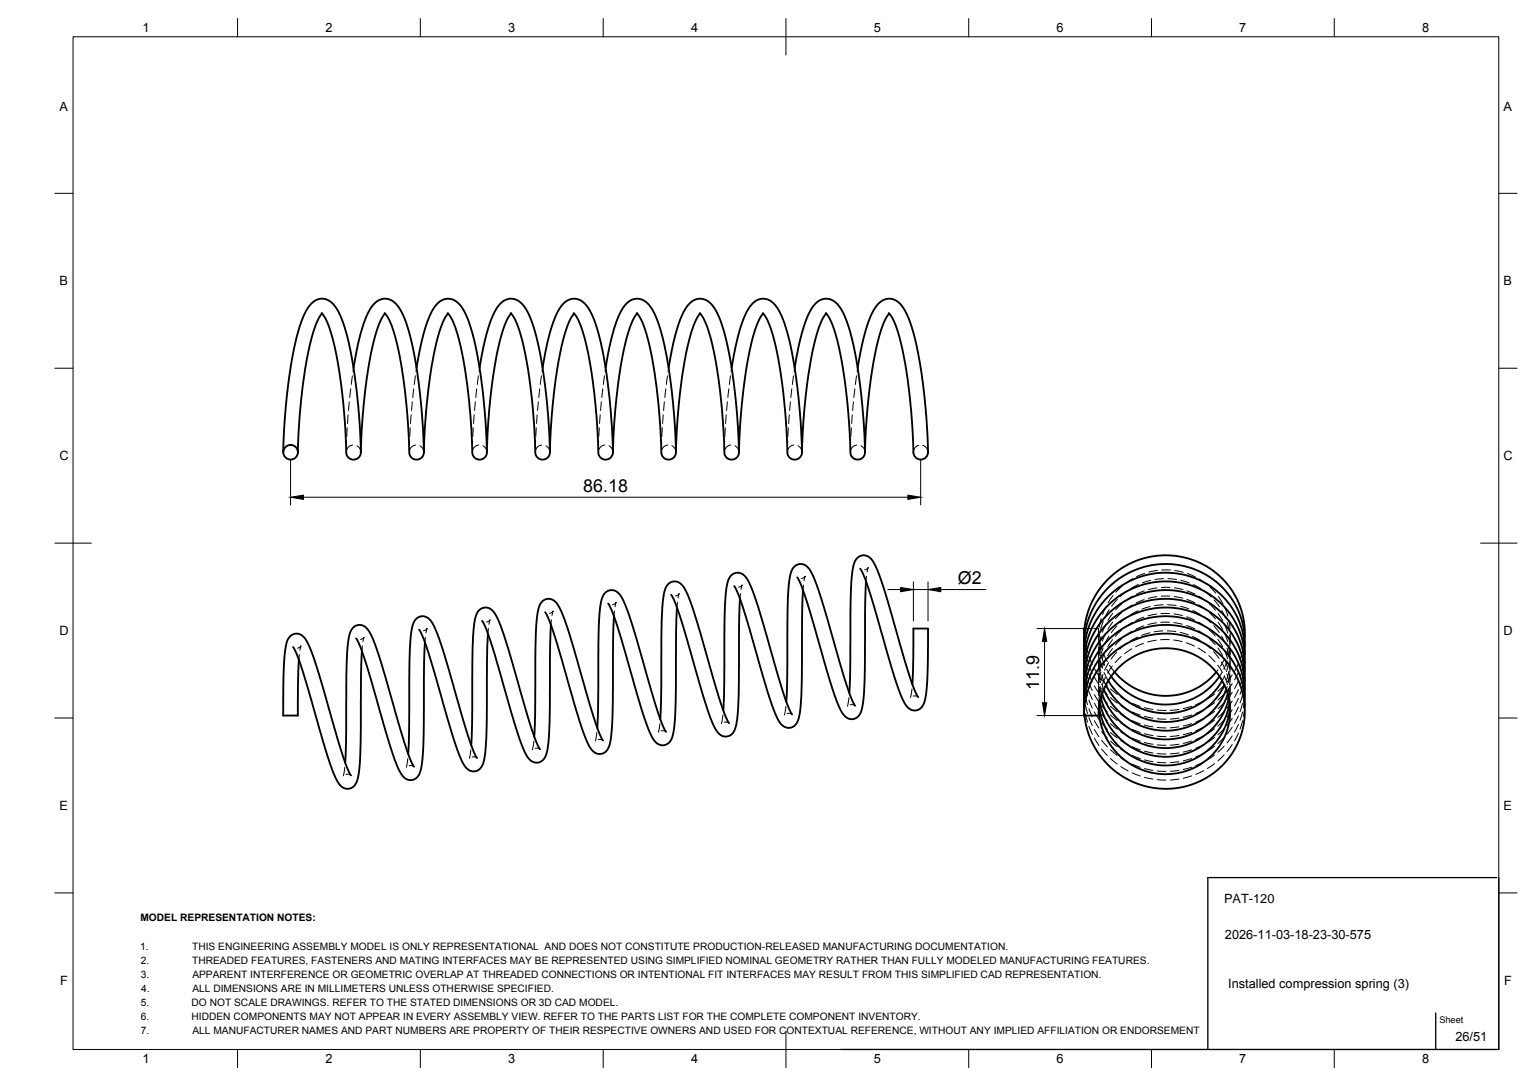
ISO-10303-21;
HEADER;
/* Generated by software containing ST-Developer
 * from STEP Tools, Inc. (www.steptools.com) 
 */

FILE_DESCRIPTION(
/* description */ ('Vibration shaker table dummy'),
/* implementation_level */ '2;1');

FILE_NAME(
/* name */ 'Installed compression spring (3).step',
/* time_stamp */ '2026-10-27T10:55:14-07:00',
/* author */ (''),
/* organization */ (''),
/* preprocessor_version */ 'ST-DEVELOPER v20.2',
/* originating_system */ 'Autodesk Translation Framework v15.17.0.0',
/* authorisation */ '');

FILE_SCHEMA (('AUTOMOTIVE_DESIGN { 1 0 10303 214 3 1 1 }'));
ENDSEC;

DATA;
#10=MECHANICAL_DESIGN_GEOMETRIC_PRESENTATION_REPRESENTATION('',(#707),#22394);
#589=B_SPLINE_CURVE_WITH_KNOTS('',3,(#20705,#20706,#20707,#20708,#20709,
#20710,#20711,#20712,#20713,#20714,#20715,#20716,#20717,#20718,#20719,#20720,
#20721,#20722,#20723,#20724,#20725,#20726,#20727,#20728,#20729,#20730,#20731,
#20732,#20733,#20734,#20735,#20736,#20737,#20738,#20739,#20740,#20741,#20742,
#20743,#20744,#20745,#20746,#20747,#20748,#20749,#20750,#20751,#20752,#20753,
#20754,#20755,#20756,#20757,#20758,#20759,#20760,#20761,#20762,#20763,#20764,
#20765,#20766,#20767,#20768,#20769,#20770,#20771,#20772,#20773,#20774,#20775,
#20776,#20777,#20778,#20779,#20780,#20781,#20782,#20783,#20784,#20785,#20786,
#20787,#20788,#20789,#20790,#20791,#20792,#20793,#20794,#20795,#20796,#20797,
#20798,#20799,#20800,#20801,#20802,#20803,#20804,#20805,#20806,#20807,#20808,
#20809,#20810,#20811,#20812,#20813,#20814,#20815,#20816,#20817,#20818,#20819,
#20820,#20821,#20822,#20823,#20824,#20825,#20826,#20827,#20828,#20829,#20830,
#20831),.UNSPECIFIED.,.F.,.F.,(4,1,1,1,1,1,1,1,1,1,1,1,1,1,1,1,1,1,1,1,
1,1,1,1,1,1,1,1,1,1,1,1,1,1,1,1,1,1,1,1,1,1,1,1,1,1,1,1,1,1,1,1,1,1,1,1,
1,1,1,1,1,1,1,1,1,1,1,1,1,1,1,1,1,1,1,1,1,1,1,1,1,1,1,1,1,1,1,1,1,1,1,1,
1,1,1,1,1,1,1,1,1,1,1,1,1,1,1,1,1,1,1,1,1,1,1,1,1,1,1,1,1,1,1,1,4),(0.,
0.00892857142857143,0.0178571428571429,0.0267857142857143,0.0357142857142857,
0.0446428571428571,0.0535714285714286,0.0625,0.0714285714285714,0.0803571428571428,
0.0892857142857143,0.0982142857142857,0.107142857142857,0.116071428571429,
0.125,0.133928571428571,0.142857142857143,0.150793650793651,0.158730158730159,
0.166666666666667,0.174603174603175,0.182539682539683,0.19047619047619,
0.196428571428571,0.202380952380952,0.208333333333333,0.214285714285714,
0.222222222222222,0.23015873015873,0.238095238095238,0.244047619047619,
0.25,0.261904761904762,0.273809523809524,0.285714285714286,0.297619047619048,
0.30952380952381,0.321428571428571,0.333333333333333,0.337301587301587,
0.341269841269841,0.349206349206349,0.357142857142857,0.365079365079365,
0.373015873015873,0.380952380952381,0.386904761904762,0.392857142857143,
0.404761904761905,0.410714285714286,0.416666666666667,0.422619047619048,
0.428571428571429,0.4375,0.446428571428571,0.455357142857143,0.459821428571429,
0.464285714285714,0.470238095238095,0.476190476190476,0.482142857142857,
0.491071428571429,0.5,0.508928571428571,0.517857142857143,0.526785714285714,
0.535714285714286,0.544642857142857,0.553571428571429,0.5625,0.571428571428571,
0.580357142857143,0.589285714285714,0.598214285714286,0.607142857142857,
0.616071428571429,0.625,0.633928571428571,0.642857142857143,0.650793650793651,
0.658730158730159,0.666666666666667,0.672619047619048,0.678571428571428,
0.684523809523809,0.69047619047619,0.696428571428571,0.702380952380952,
0.708333333333333,0.714285714285714,0.720238095238095,0.726190476190476,
0.732142857142857,0.738095238095238,0.744047619047619,0.75,0.755952380952381,
0.761904761904762,0.76984126984127,0.777777777777778,0.785714285714286,
0.794642857142857,0.803571428571428,0.8125,0.821428571428571,0.830357142857143,
0.839285714285714,0.848214285714286,0.857142857142857,0.866071428571429,
0.875,0.883928571428571,0.892857142857143,0.901785714285714,0.910714285714286,
0.919642857142857,0.928571428571429,0.9375,0.946428571428571,0.955357142857143,
0.964285714285714,0.973214285714286,0.982142857142857,0.991071428571429,
1.),.UNSPECIFIED.);
#593=B_SPLINE_SURFACE_WITH_KNOTS('',3,3,((#19432,#19433,#19434,#19435,#19436,
#19437,#19438,#19439,#19440,#19441,#19442,#19443,#19444,#19445,#19446,#19447,
#19448,#19449,#19450,#19451,#19452,#19453,#19454,#19455,#19456,#19457,#19458,
#19459,#19460,#19461,#19462,#19463,#19464,#19465,#19466,#19467,#19468,#19469,
#19470,#19471,#19472,#19473,#19474,#19475,#19476,#19477,#19478,#19479,#19480,
#19481,#19482,#19483,#19484,#19485,#19486,#19487,#19488,#19489,#19490,#19491,
#19492,#19493,#19494,#19495,#19496,#19497,#19498,#19499,#19500,#19501,#19502,
#19503,#19504,#19505,#19506,#19507,#19508,#19509,#19510,#19511,#19512,#19513,
#19514,#19515,#19516,#19517,#19518,#19519,#19520,#19521,#19522,#19523,#19524,
#19525,#19526,#19527,#19528,#19529,#19530,#19531,#19532,#19533,#19534,#19535,
#19536,#19537,#19538,#19539,#19540,#19541,#19542,#19543,#19544,#19545,#19546,
#19547,#19548,#19549,#19550,#19551,#19552,#19553,#19554,#19555,#19556,#19557,
#19558),(#19559,#19560,#19561,#19562,#19563,#19564,#19565,#19566,#19567,
#19568,#19569,#19570,#19571,#19572,#19573,#19574,#19575,#19576,#19577,#19578,
#19579,#19580,#19581,#19582,#19583,#19584,#19585,#19586,#19587,#19588,#19589,
#19590,#19591,#19592,#19593,#19594,#19595,#19596,#19597,#19598,#19599,#19600,
#19601,#19602,#19603,#19604,#19605,#19606,#19607,#19608,#19609,#19610,#19611,
#19612,#19613,#19614,#19615,#19616,#19617,#19618,#19619,#19620,#19621,#19622,
#19623,#19624,#19625,#19626,#19627,#19628,#19629,#19630,#19631,#19632,#19633,
#19634,#19635,#19636,#19637,#19638,#19639,#19640,#19641,#19642,#19643,#19644,
#19645,#19646,#19647,#19648,#19649,#19650,#19651,#19652,#19653,#19654,#19655,
#19656,#19657,#19658,#19659,#19660,#19661,#19662,#19663,#19664,#19665,#19666,
#19667,#19668,#19669,#19670,#19671,#19672,#19673,#19674,#19675,#19676,#19677,
#19678,#19679,#19680,#19681,#19682,#19683,#19684,#19685),(#19686,#19687,
#19688,#19689,#19690,#19691,#19692,#19693,#19694,#19695,#19696,#19697,#19698,
#19699,#19700,#19701,#19702,#19703,#19704,#19705,#19706,#19707,#19708,#19709,
#19710,#19711,#19712,#19713,#19714,#19715,#19716,#19717,#19718,#19719,#19720,
#19721,#19722,#19723,#19724,#19725,#19726,#19727,#19728,#19729,#19730,#19731,
#19732,#19733,#19734,#19735,#19736,#19737,#19738,#19739,#19740,#19741,#19742,
#19743,#19744,#19745,#19746,#19747,#19748,#19749,#19750,#19751,#19752,#19753,
#19754,#19755,#19756,#19757,#19758,#19759,#19760,#19761,#19762,#19763,#19764,
#19765,#19766,#19767,#19768,#19769,#19770,#19771,#19772,#19773,#19774,#19775,
#19776,#19777,#19778,#19779,#19780,#19781,#19782,#19783,#19784,#19785,#19786,
#19787,#19788,#19789,#19790,#19791,#19792,#19793,#19794,#19795,#19796,#19797,
#19798,#19799,#19800,#19801,#19802,#19803,#19804,#19805,#19806,#19807,#19808,
#19809,#19810,#19811,#19812),(#19813,#19814,#19815,#19816,#19817,#19818,
#19819,#19820,#19821,#19822,#19823,#19824,#19825,#19826,#19827,#19828,#19829,
#19830,#19831,#19832,#19833,#19834,#19835,#19836,#19837,#19838,#19839,#19840,
#19841,#19842,#19843,#19844,#19845,#19846,#19847,#19848,#19849,#19850,#19851,
#19852,#19853,#19854,#19855,#19856,#19857,#19858,#19859,#19860,#19861,#19862,
#19863,#19864,#19865,#19866,#19867,#19868,#19869,#19870,#19871,#19872,#19873,
#19874,#19875,#19876,#19877,#19878,#19879,#19880,#19881,#19882,#19883,#19884,
#19885,#19886,#19887,#19888,#19889,#19890,#19891,#19892,#19893,#19894,#19895,
#19896,#19897,#19898,#19899,#19900,#19901,#19902,#19903,#19904,#19905,#19906,
#19907,#19908,#19909,#19910,#19911,#19912,#19913,#19914,#19915,#19916,#19917,
#19918,#19919,#19920,#19921,#19922,#19923,#19924,#19925,#19926,#19927,#19928,
#19929,#19930,#19931,#19932,#19933,#19934,#19935,#19936,#19937,#19938,#19939),
(#19940,#19941,#19942,#19943,#19944,#19945,#19946,#19947,#19948,#19949,
#19950,#19951,#19952,#19953,#19954,#19955,#19956,#19957,#19958,#19959,#19960,
#19961,#19962,#19963,#19964,#19965,#19966,#19967,#19968,#19969,#19970,#19971,
#19972,#19973,#19974,#19975,#19976,#19977,#19978,#19979,#19980,#19981,#19982,
#19983,#19984,#19985,#19986,#19987,#19988,#19989,#19990,#19991,#19992,#19993,
#19994,#19995,#19996,#19997,#19998,#19999,#20000,#20001,#20002,#20003,#20004,
#20005,#20006,#20007,#20008,#20009,#20010,#20011,#20012,#20013,#20014,#20015,
#20016,#20017,#20018,#20019,#20020,#20021,#20022,#20023,#20024,#20025,#20026,
#20027,#20028,#20029,#20030,#20031,#20032,#20033,#20034,#20035,#20036,#20037,
#20038,#20039,#20040,#20041,#20042,#20043,#20044,#20045,#20046,#20047,#20048,
#20049,#20050,#20051,#20052,#20053,#20054,#20055,#20056,#20057,#20058,#20059,
#20060,#20061,#20062,#20063,#20064,#20065,#20066),(#20067,#20068,#20069,
#20070,#20071,#20072,#20073,#20074,#20075,#20076,#20077,#20078,#20079,#20080,
#20081,#20082,#20083,#20084,#20085,#20086,#20087,#20088,#20089,#20090,#20091,
#20092,#20093,#20094,#20095,#20096,#20097,#20098,#20099,#20100,#20101,#20102,
#20103,#20104,#20105,#20106,#20107,#20108,#20109,#20110,#20111,#20112,#20113,
#20114,#20115,#20116,#20117,#20118,#20119,#20120,#20121,#20122,#20123,#20124,
#20125,#20126,#20127,#20128,#20129,#20130,#20131,#20132,#20133,#20134,#20135,
#20136,#20137,#20138,#20139,#20140,#20141,#20142,#20143,#20144,#20145,#20146,
#20147,#20148,#20149,#20150,#20151,#20152,#20153,#20154,#20155,#20156,#20157,
#20158,#20159,#20160,#20161,#20162,#20163,#20164,#20165,#20166,#20167,#20168,
#20169,#20170,#20171,#20172,#20173,#20174,#20175,#20176,#20177,#20178,#20179,
#20180,#20181,#20182,#20183,#20184,#20185,#20186,#20187,#20188,#20189,#20190,
#20191,#20192,#20193),(#20194,#20195,#20196,#20197,#20198,#20199,#20200,
#20201,#20202,#20203,#20204,#20205,#20206,#20207,#20208,#20209,#20210,#20211,
#20212,#20213,#20214,#20215,#20216,#20217,#20218,#20219,#20220,#20221,#20222,
#20223,#20224,#20225,#20226,#20227,#20228,#20229,#20230,#20231,#20232,#20233,
#20234,#20235,#20236,#20237,#20238,#20239,#20240,#20241,#20242,#20243,#20244,
#20245,#20246,#20247,#20248,#20249,#20250,#20251,#20252,#20253,#20254,#20255,
#20256,#20257,#20258,#20259,#20260,#20261,#20262,#20263,#20264,#20265,#20266,
#20267,#20268,#20269,#20270,#20271,#20272,#20273,#20274,#20275,#20276,#20277,
#20278,#20279,#20280,#20281,#20282,#20283,#20284,#20285,#20286,#20287,#20288,
#20289,#20290,#20291,#20292,#20293,#20294,#20295,#20296,#20297,#20298,#20299,
#20300,#20301,#20302,#20303,#20304,#20305,#20306,#20307,#20308,#20309,#20310,
#20311,#20312,#20313,#20314,#20315,#20316,#20317,#20318,#20319,#20320),
(#20321,#20322,#20323,#20324,#20325,#20326,#20327,#20328,#20329,#20330,
#20331,#20332,#20333,#20334,#20335,#20336,#20337,#20338,#20339,#20340,#20341,
#20342,#20343,#20344,#20345,#20346,#20347,#20348,#20349,#20350,#20351,#20352,
#20353,#20354,#20355,#20356,#20357,#20358,#20359,#20360,#20361,#20362,#20363,
#20364,#20365,#20366,#20367,#20368,#20369,#20370,#20371,#20372,#20373,#20374,
#20375,#20376,#20377,#20378,#20379,#20380,#20381,#20382,#20383,#20384,#20385,
#20386,#20387,#20388,#20389,#20390,#20391,#20392,#20393,#20394,#20395,#20396,
#20397,#20398,#20399,#20400,#20401,#20402,#20403,#20404,#20405,#20406,#20407,
#20408,#20409,#20410,#20411,#20412,#20413,#20414,#20415,#20416,#20417,#20418,
#20419,#20420,#20421,#20422,#20423,#20424,#20425,#20426,#20427,#20428,#20429,
#20430,#20431,#20432,#20433,#20434,#20435,#20436,#20437,#20438,#20439,#20440,
#20441,#20442,#20443,#20444,#20445,#20446,#20447),(#20448,#20449,#20450,
#20451,#20452,#20453,#20454,#20455,#20456,#20457,#20458,#20459,#20460,#20461,
#20462,#20463,#20464,#20465,#20466,#20467,#20468,#20469,#20470,#20471,#20472,
#20473,#20474,#20475,#20476,#20477,#20478,#20479,#20480,#20481,#20482,#20483,
#20484,#20485,#20486,#20487,#20488,#20489,#20490,#20491,#20492,#20493,#20494,
#20495,#20496,#20497,#20498,#20499,#20500,#20501,#20502,#20503,#20504,#20505,
#20506,#20507,#20508,#20509,#20510,#20511,#20512,#20513,#20514,#20515,#20516,
#20517,#20518,#20519,#20520,#20521,#20522,#20523,#20524,#20525,#20526,#20527,
#20528,#20529,#20530,#20531,#20532,#20533,#20534,#20535,#20536,#20537,#20538,
#20539,#20540,#20541,#20542,#20543,#20544,#20545,#20546,#20547,#20548,#20549,
#20550,#20551,#20552,#20553,#20554,#20555,#20556,#20557,#20558,#20559,#20560,
#20561,#20562,#20563,#20564,#20565,#20566,#20567,#20568,#20569,#20570,#20571,
#20572,#20573,#20574),(#20575,#20576,#20577,#20578,#20579,#20580,#20581,
#20582,#20583,#20584,#20585,#20586,#20587,#20588,#20589,#20590,#20591,#20592,
#20593,#20594,#20595,#20596,#20597,#20598,#20599,#20600,#20601,#20602,#20603,
#20604,#20605,#20606,#20607,#20608,#20609,#20610,#20611,#20612,#20613,#20614,
#20615,#20616,#20617,#20618,#20619,#20620,#20621,#20622,#20623,#20624,#20625,
#20626,#20627,#20628,#20629,#20630,#20631,#20632,#20633,#20634,#20635,#20636,
#20637,#20638,#20639,#20640,#20641,#20642,#20643,#20644,#20645,#20646,#20647,
#20648,#20649,#20650,#20651,#20652,#20653,#20654,#20655,#20656,#20657,#20658,
#20659,#20660,#20661,#20662,#20663,#20664,#20665,#20666,#20667,#20668,#20669,
#20670,#20671,#20672,#20673,#20674,#20675,#20676,#20677,#20678,#20679,#20680,
#20681,#20682,#20683,#20684,#20685,#20686,#20687,#20688,#20689,#20690,#20691,
#20692,#20693,#20694,#20695,#20696,#20697,#20698,#20699,#20700,#20701)),
 .UNSPECIFIED.,.T.,.F.,.F.,(4,1,1,1,1,1,1,4),(4,1,1,1,1,1,1,1,1,1,1,1,1,
1,1,1,1,1,1,1,1,1,1,1,1,1,1,1,1,1,1,1,1,1,1,1,1,1,1,1,1,1,1,1,1,1,1,1,1,
1,1,1,1,1,1,1,1,1,1,1,1,1,1,1,1,1,1,1,1,1,1,1,1,1,1,1,1,1,1,1,1,1,1,1,1,
1,1,1,1,1,1,1,1,1,1,1,1,1,1,1,1,1,1,1,1,1,1,1,1,1,1,1,1,1,1,1,1,1,1,1,1,
1,1,1,4),(-3.14159265358979,-2.24399475256414,-1.34639685153848,-0.448798950512828,
0.448798950512828,1.34639685153848,2.24399475256414,3.14159265358979),(0.,
0.00892857142857143,0.0178571428571429,0.0267857142857143,0.0357142857142857,
0.0446428571428571,0.0535714285714286,0.0625,0.0714285714285714,0.0803571428571428,
0.0892857142857143,0.0982142857142857,0.107142857142857,0.116071428571429,
0.125,0.133928571428571,0.142857142857143,0.150793650793651,0.158730158730159,
0.166666666666667,0.174603174603175,0.182539682539683,0.19047619047619,
0.196428571428571,0.202380952380952,0.208333333333333,0.214285714285714,
0.222222222222222,0.23015873015873,0.238095238095238,0.244047619047619,
0.25,0.261904761904762,0.273809523809524,0.285714285714286,0.297619047619048,
0.30952380952381,0.321428571428571,0.333333333333333,0.337301587301587,
0.341269841269841,0.349206349206349,0.357142857142857,0.365079365079365,
0.373015873015873,0.380952380952381,0.386904761904762,0.392857142857143,
0.404761904761905,0.410714285714286,0.416666666666667,0.422619047619048,
0.428571428571429,0.4375,0.446428571428571,0.455357142857143,0.459821428571429,
0.464285714285714,0.470238095238095,0.476190476190476,0.482142857142857,
0.491071428571429,0.5,0.508928571428571,0.517857142857143,0.526785714285714,
0.535714285714286,0.544642857142857,0.553571428571429,0.5625,0.571428571428571,
0.580357142857143,0.589285714285714,0.598214285714286,0.607142857142857,
0.616071428571429,0.625,0.633928571428571,0.642857142857143,0.650793650793651,
0.658730158730159,0.666666666666667,0.672619047619048,0.678571428571428,
0.684523809523809,0.69047619047619,0.696428571428571,0.702380952380952,
0.708333333333333,0.714285714285714,0.720238095238095,0.726190476190476,
0.732142857142857,0.738095238095238,0.744047619047619,0.75,0.755952380952381,
0.761904761904762,0.76984126984127,0.777777777777778,0.785714285714286,
0.794642857142857,0.803571428571428,0.8125,0.821428571428571,0.830357142857143,
0.839285714285714,0.848214285714286,0.857142857142857,0.866071428571429,
0.875,0.883928571428571,0.892857142857143,0.901785714285714,0.910714285714286,
0.919642857142857,0.928571428571429,0.9375,0.946428571428571,0.955357142857143,
0.964285714285714,0.973214285714286,0.982142857142857,0.991071428571429,
1.),.UNSPECIFIED.);
#615=SHAPE_REPRESENTATION_RELATIONSHIP('SRR','None',#22661,#661);
#661=ADVANCED_BREP_SHAPE_REPRESENTATION('',(#753),#22367);
#707=STYLED_ITEM('',(#22961),#753);
#753=MANIFOLD_SOLID_BREP('Body1',#9225);
#1190=PLANE('',#10202);
#1191=PLANE('',#10203);
#1562=FACE_OUTER_BOUND('',#2204,.T.);
#1563=FACE_OUTER_BOUND('',#2205,.T.);
#1564=FACE_OUTER_BOUND('',#2206,.T.);
#2204=EDGE_LOOP('',(#7272,#7273,#7274,#7275));
#2205=EDGE_LOOP('',(#7276));
#2206=EDGE_LOOP('',(#7277));
#4058=CIRCLE('',#10200,0.1);
#4059=CIRCLE('',#10201,0.1);
#4709=VERTEX_POINT('',#20702);
#4710=VERTEX_POINT('',#20704);
#5629=EDGE_CURVE('',#4709,#4709,#4058,.T.);
#5630=EDGE_CURVE('',#4709,#4710,#589,.T.);
#5631=EDGE_CURVE('',#4710,#4710,#4059,.T.);
#7272=ORIENTED_EDGE('',*,*,#5629,.T.);
#7273=ORIENTED_EDGE('',*,*,#5630,.T.);
#7274=ORIENTED_EDGE('',*,*,#5631,.F.);
#7275=ORIENTED_EDGE('',*,*,#5630,.F.);
#7276=ORIENTED_EDGE('',*,*,#5631,.T.);
#7277=ORIENTED_EDGE('',*,*,#5629,.F.);
#8927=ADVANCED_FACE('',(#1562),#593,.T.);
#8928=ADVANCED_FACE('',(#1563),#1190,.T.);
#8929=ADVANCED_FACE('',(#1564),#1191,.F.);
#9225=CLOSED_SHELL('',(#8927,#8928,#8929));
#10199=AXIS2_PLACEMENT_3D('',#19431,#12140,#12141);
#10200=AXIS2_PLACEMENT_3D('',#20703,#12142,#12143);
#10201=AXIS2_PLACEMENT_3D('',#20832,#12144,#12145);
#10202=AXIS2_PLACEMENT_3D('',#20833,#12146,#12147);
#10203=AXIS2_PLACEMENT_3D('',#20834,#12148,#12149);
#12140=DIRECTION('axis',(0.,0.,1.));
#12141=DIRECTION('refdir',(1.,0.,0.));
#12142=DIRECTION('center_axis',(-0.000133356251592195,0.990604928516511,
0.136754735987128));
#12143=DIRECTION('ref_axis',(1.84100626682885E-5,-0.136754734747938,0.990604937492788));
#12144=DIRECTION('center_axis',(0.000133356514576091,0.990604928496106,
0.136754736134679));
#12145=DIRECTION('ref_axis',(-0.72222669792222,0.0946826992558859,-0.685145081913302));
#12146=DIRECTION('center_axis',(0.000133356514576091,0.990604928496106,
0.136754736134679));
#12147=DIRECTION('ref_axis',(-0.72222669792222,0.0946826992558859,-0.685145081913302));
#12148=DIRECTION('center_axis',(-0.000133356251592195,0.990604928516511,
0.136754735987128));
#12149=DIRECTION('ref_axis',(1.84100626682885E-5,-0.136754734747938,0.990604937492788));
#19431=CARTESIAN_POINT('',(0.,0.,0.));
#19432=CARTESIAN_POINT('Ctrl Pts',(6.99999815899373,4.01367547347479,2.60093950625072));
#19433=CARTESIAN_POINT('Ctrl Pts',(6.99997288064589,4.20144961727953,2.62686205390015));
#19434=CARTESIAN_POINT('Ctrl Pts',(6.89230845853935,4.57620131355266,2.67882572810781));
#19435=CARTESIAN_POINT('Ctrl Pts',(6.45268902055693,4.97011892113672,2.75738771144581));
#19436=CARTESIAN_POINT('Ctrl Pts',(5.86669155617951,5.07009441973235,2.83651805910941));
#19437=CARTESIAN_POINT('Ctrl Pts',(5.31323924231124,4.84148977638369,2.91622570222972));
#19438=CARTESIAN_POINT('Ctrl Pts',(4.96382442320151,4.34995448969575,2.99649058141579));
#19439=CARTESIAN_POINT('Ctrl Pts',(4.92922815468166,3.74381008719936,3.07730076310524));
#19440=CARTESIAN_POINT('Ctrl Pts',(5.22433988671615,3.20870475874992,3.15863604084508));
#19441=CARTESIAN_POINT('Ctrl Pts',(5.76222017520179,2.91082295270622,3.24047540691231));
#19442=CARTESIAN_POINT('Ctrl Pts',(6.37972244802771,2.94499376197989,3.3227938596108));
#19443=CARTESIAN_POINT('Ctrl Pts',(6.88714214280083,3.30444617999842,3.40556405334158));
#19444=CARTESIAN_POINT('Ctrl Pts',(7.1267179261553,3.88170395597293,3.48875576611263));
#19445=CARTESIAN_POINT('Ctrl Pts',(7.02193956541344,4.50081591971197,3.57233637082151));
#19446=CARTESIAN_POINT('Ctrl Pts',(6.60200309921583,4.97124649007052,3.65627092163634));
#19447=CARTESIAN_POINT('Ctrl Pts',(5.99391816782283,5.1467637293928,3.74052239101179));
#19448=CARTESIAN_POINT('Ctrl Pts',(5.38351410020794,4.97125258500565,3.82505187835831));
#19449=CARTESIAN_POINT('Ctrl Pts',(4.97495278641361,4.51407471129711,3.90667930564871));
#19450=CARTESIAN_POINT('Ctrl Pts',(4.85890493436876,3.9395318134167,3.98533819655606));
#19451=CARTESIAN_POINT('Ctrl Pts',(5.0248445336464,3.40104453051283,4.06097495851984));
#19452=CARTESIAN_POINT('Ctrl Pts',(5.42877344681216,3.00706135834947,4.13670514776413));
#19453=CARTESIAN_POINT('Ctrl Pts',(5.97224138292893,2.85377277882407,4.21249751166765));
#19454=CARTESIAN_POINT('Ctrl Pts',(6.52306794486814,2.97976887786423,4.28832050304671));
#19455=CARTESIAN_POINT('Ctrl Pts',(6.911106619782,3.32248792481664,4.35782394345616));
#19456=CARTESIAN_POINT('Ctrl Pts',(7.09651656274147,3.74815778477591,4.4209850314008));
#19457=CARTESIAN_POINT('Ctrl Pts',(7.11222142726568,4.16541427135673,4.47779829351342));
#19458=CARTESIAN_POINT('Ctrl Pts',(6.97427650626816,4.55914085431083,4.53456660987697));
#19459=CARTESIAN_POINT('Ctrl Pts',(6.6723790417336,4.91046294860728,4.59757802409045));
#19460=CARTESIAN_POINT('Ctrl Pts',(6.20229995228089,5.12240612151564,4.66678931423933));
#19461=CARTESIAN_POINT('Ctrl Pts',(5.6425500433818,5.08009523000915,4.74213609069821));
#19462=CARTESIAN_POINT('Ctrl Pts',(5.21136094690014,4.8013569526932,4.8110335703418));
#19463=CARTESIAN_POINT('Ctrl Pts',(4.96782069609662,4.41239190726546,4.87351124705845));
#19464=CARTESIAN_POINT('Ctrl Pts',(4.86407127402864,3.87207825314686,4.94830807657783));
#19465=CARTESIAN_POINT('Ctrl Pts',(5.12715288076494,3.20107434287668,5.041444793684));
#19466=CARTESIAN_POINT('Ctrl Pts',(5.90376531288412,2.82823955973182,5.15254762811187));
#19467=CARTESIAN_POINT('Ctrl Pts',(6.72029013273465,3.08146453910134,5.2629101070658));
#19468=CARTESIAN_POINT('Ctrl Pts',(7.14364665428008,3.81715099008766,5.37246078991918));
#19469=CARTESIAN_POINT('Ctrl Pts',(6.9551205530812,4.63769652624648,5.4811367937548));
#19470=CARTESIAN_POINT('Ctrl Pts',(6.2641024490546,5.1069317667711,5.5888844628491));
#19471=CARTESIAN_POINT('Ctrl Pts',(5.62881174521816,5.00949357808685,5.67193196549233));
#19472=CARTESIAN_POINT('Ctrl Pts',(5.2874560242671,4.74926815537235,5.73087908447157));
#19473=CARTESIAN_POINT('Ctrl Pts',(5.07381541095866,4.48213637560843,5.77788659685938));
#19474=CARTESIAN_POINT('Ctrl Pts',(4.94552168624609,4.06557538718633,5.83636209008294));
#19475=CARTESIAN_POINT('Ctrl Pts',(5.04911869155687,3.55670415977292,5.90607316299982));
#19476=CARTESIAN_POINT('Ctrl Pts',(5.38099173791495,3.16160536520236,5.97532164753646));
#19477=CARTESIAN_POINT('Ctrl Pts',(5.85816561666817,2.97493727370523,6.04410657341625));
#19478=CARTESIAN_POINT('Ctrl Pts',(6.32119024886796,3.03347138881056,6.1067356435835));
#19479=CARTESIAN_POINT('Ctrl Pts',(6.67264815667528,3.25520245847479,6.16333652453463));
#19480=CARTESIAN_POINT('Ctrl Pts',(6.9689172446974,3.65479400388877,6.23091649769543));
#19481=CARTESIAN_POINT('Ctrl Pts',(7.0079089842411,4.17131843581214,6.29799027327548));
#19482=CARTESIAN_POINT('Ctrl Pts',(6.77691391923214,4.60388596675421,6.36457330679182));
#19483=CARTESIAN_POINT('Ctrl Pts',(6.50054973430609,4.84205531318333,6.414270318429));
#19484=CARTESIAN_POINT('Ctrl Pts',(6.15708960805529,4.96183696463414,6.46373244636263));
#19485=CARTESIAN_POINT('Ctrl Pts',(5.73515865256543,4.94625066250657,6.52117144063107));
#19486=CARTESIAN_POINT('Ctrl Pts',(5.30609465295405,4.70907742816445,6.5864458994691));
#19487=CARTESIAN_POINT('Ctrl Pts',(5.04126574291307,4.22881801076535,6.65940509117474));
#19488=CARTESIAN_POINT('Ctrl Pts',(5.06730780646012,3.7758858483265,6.71983222415362));
#19489=CARTESIAN_POINT('Ctrl Pts',(5.22892555890349,3.46412922360998,6.7679659145206));
#19490=CARTESIAN_POINT('Ctrl Pts',(5.4292015128227,3.25210405867328,6.80796630929891));
#19491=CARTESIAN_POINT('Ctrl Pts',(5.71433691472614,3.10148200562693,6.85183024183257));
#19492=CARTESIAN_POINT('Ctrl Pts',(6.06256514105404,3.06238687711817,6.89952195897341));
#19493=CARTESIAN_POINT('Ctrl Pts',(6.4564976195634,3.16770820022483,6.95498839068538));
#19494=CARTESIAN_POINT('Ctrl Pts',(6.8102288164166,3.48372159458398,7.01814871427154));
#19495=CARTESIAN_POINT('Ctrl Pts',(6.95714247630162,3.9949743218129,7.08893288176131));
#19496=CARTESIAN_POINT('Ctrl Pts',(6.81021696910949,4.50416338125004,7.1594866624322));
#19497=CARTESIAN_POINT('Ctrl Pts',(6.41591912974157,4.85632155826513,7.22985222666365));
#19498=CARTESIAN_POINT('Ctrl Pts',(5.89581150258709,4.9445435848153,7.30007283488175));
#19499=CARTESIAN_POINT('Ctrl Pts',(5.4091541149686,4.74288106481787,7.37019262264602));
#19500=CARTESIAN_POINT('Ctrl Pts',(5.1045916955003,4.31357351873737,7.4402563254929));
#19501=CARTESIAN_POINT('Ctrl Pts',(5.07507074796588,3.78812027671986,7.51030900575102));
#19502=CARTESIAN_POINT('Ctrl Pts',(5.32971571962661,3.32725097083008,7.58039577698861));
#19503=CARTESIAN_POINT('Ctrl Pts',(5.79102376728976,3.07217291555275,7.65056157443439));
#19504=CARTESIAN_POINT('Ctrl Pts',(6.31826217852957,3.10162768020774,7.72085085716367));
#19505=CARTESIAN_POINT('Ctrl Pts',(6.75007083293795,3.40776502742426,7.79130734598018));
#19506=CARTESIAN_POINT('Ctrl Pts',(6.95345754831281,3.89815513784294,7.86197377424134));
#19507=CARTESIAN_POINT('Ctrl Pts',(6.86450758322969,4.42345798565047,7.9328916442996));
#19508=CARTESIAN_POINT('Ctrl Pts',(6.50825373195115,4.82258144361629,8.00410096577401));
#19509=CARTESIAN_POINT('Ctrl Pts',(5.99196133471143,4.97171282731416,8.07564000535001));
#19510=CARTESIAN_POINT('Ctrl Pts',(5.47264846544098,4.82257977354425,8.14754510597589));
#19511=CARTESIAN_POINT('Ctrl Pts',(5.12402089676511,4.43277938176583,8.21717246163365));
#19512=CARTESIAN_POINT('Ctrl Pts',(5.02434526751946,3.94102818280025,8.28449961898673));
#19513=CARTESIAN_POINT('Ctrl Pts',(5.16694197219437,3.47827882962972,8.34949563910625));
#19514=CARTESIAN_POINT('Ctrl Pts',(5.48619587513468,3.16623898773365,8.40942447363167));
#19515=CARTESIAN_POINT('Ctrl Pts',(5.86631955340104,3.03340212556353,8.46419547601151));
#19516=CARTESIAN_POINT('Ctrl Pts',(6.22999033724363,3.04672408117636,8.5137197912885));
#19517=CARTESIAN_POINT('Ctrl Pts',(6.56525962631825,3.19292643023923,8.5634804916257));
#19518=CARTESIAN_POINT('Ctrl Pts',(6.82522778577244,3.45264122124887,8.61348288970028));
#19519=CARTESIAN_POINT('Ctrl Pts',(6.97307814435936,3.7910761621246,8.66373168303779));
#19520=CARTESIAN_POINT('Ctrl Pts',(6.98712736643486,4.16195247500926,8.71423091450252));
#19521=CARTESIAN_POINT('Ctrl Pts',(6.86409623902891,4.5140922960367,8.76498396821101));
#19522=CARTESIAN_POINT('Ctrl Pts',(6.61968565405262,4.79836651831856,8.81599356006379));
#19523=CARTESIAN_POINT('Ctrl Pts',(6.28663324217223,4.97458782653242,8.86726173278701));
#19524=CARTESIAN_POINT('Ctrl Pts',(5.9103163648716,5.01715912899264,8.91878984727219));
#19525=CARTESIAN_POINT('Ctrl Pts',(5.5426151162157,4.91881558382611,8.97057858184767));
#19526=CARTESIAN_POINT('Ctrl Pts',(5.2346932137367,4.69177671709244,9.02262792714338));
#19527=CARTESIAN_POINT('Ctrl Pts',(5.03002927873253,4.36635777160092,9.07493719269484));
#19528=CARTESIAN_POINT('Ctrl Pts',(4.95793528493379,3.98670141138964,9.12750499446544));
#19529=CARTESIAN_POINT('Ctrl Pts',(5.03011221582078,3.60530312678215,9.18032928985668));
#19530=CARTESIAN_POINT('Ctrl Pts',(5.26028491013977,3.23792219176526,9.23930487837506));
#19531=CARTESIAN_POINT('Ctrl Pts',(5.66833767471456,2.97390330572424,9.30453505298122));
#19532=CARTESIAN_POINT('Ctrl Pts',(6.20020835504347,2.93396150339657,9.37613052320119));
#19533=CARTESIAN_POINT('Ctrl Pts',(6.70998344550478,3.16323515745987,9.45115011118038));
#19534=CARTESIAN_POINT('Ctrl Pts',(7.05174463296735,3.64363058779886,9.52964181253653));
#19535=CARTESIAN_POINT('Ctrl Pts',(7.08674491429888,4.25878461683797,9.61164803498578));
#19536=CARTESIAN_POINT('Ctrl Pts',(6.78746221281555,4.80126791369132,9.69412424256602));
#19537=CARTESIAN_POINT('Ctrl Pts',(6.24245359179364,5.10299460367291,9.77704205650278));
#19538=CARTESIAN_POINT('Ctrl Pts',(5.617389337803,5.06829072683056,9.86037045574097));
#19539=CARTESIAN_POINT('Ctrl Pts',(5.10428990247565,4.70469241242162,9.94407602255943));
#19540=CARTESIAN_POINT('Ctrl Pts',(4.86233610468105,4.12145238678417,10.0281230884956));
#19541=CARTESIAN_POINT('Ctrl Pts',(4.96818752346366,3.49664100367693,10.1124739581892));
#19542=CARTESIAN_POINT('Ctrl Pts',(5.39158733307429,3.02246211865203,10.197089152739));
#19543=CARTESIAN_POINT('Ctrl Pts',(6.00398991824946,2.84580444666258,10.2819276236503));
#19544=CARTESIAN_POINT('Ctrl Pts',(6.61780477214459,3.0224619351938,10.3669470022194));
#19545=CARTESIAN_POINT('Ctrl Pts',(7.04420003577297,3.49941215707345,10.4521038303345));
#19546=CARTESIAN_POINT('Ctrl Pts',(7.15155414725,4.13081128487796,10.5373538665558));
#19547=CARTESIAN_POINT('Ctrl Pts',(6.90634183228622,4.72286458915024,10.6226522963591));
#19548=CARTESIAN_POINT('Ctrl Pts',(6.38367034420738,5.09368398946472,10.7079540131199));
#19549=CARTESIAN_POINT('Ctrl Pts',(5.74412845724406,5.12951897848491,10.7932138931513));
#19550=CARTESIAN_POINT('Ctrl Pts',(5.18413119725411,4.81987766303419,10.8783870658711));
#19551=CARTESIAN_POINT('Ctrl Pts',(4.8752129919825,4.26058851376116,10.9634291554075));
#19552=CARTESIAN_POINT('Ctrl Pts',(4.91115871222138,3.62399076997319,11.0482965295163));
#19553=CARTESIAN_POINT('Ctrl Pts',(5.27935908785992,3.10540850794678,11.1329466617017));
#19554=CARTESIAN_POINT('Ctrl Pts',(5.86521072908837,2.86304864268273,11.2173381122335));
#19555=CARTESIAN_POINT('Ctrl Pts',(6.48796989668153,2.969020134583,11.3014313415043));
#19556=CARTESIAN_POINT('Ctrl Pts',(6.95689206969945,3.38875839075872,11.3851878190745));
#19557=CARTESIAN_POINT('Ctrl Pts',(7.07219562678887,3.7896496622666,11.4407823887692));
#19558=CARTESIAN_POINT('Ctrl Pts',(7.07222266979222,3.99053173007441,11.4685145081913));
#19559=CARTESIAN_POINT('Ctrl Pts',(6.97007822923066,4.01367144562316,2.60093950625072));
#19560=CARTESIAN_POINT('Ctrl Pts',(6.97005368434554,4.19599723746873,2.62610989942131));
#19561=CARTESIAN_POINT('Ctrl Pts',(6.86557136883425,4.55976104448084,2.67654110363146));
#19562=CARTESIAN_POINT('Ctrl Pts',(6.43865008190508,4.94238932286108,2.75283713480025));
#19563=CARTESIAN_POINT('Ctrl Pts',(5.86921493316712,5.03959284630734,2.82972340130287));
#19564=CARTESIAN_POINT('Ctrl Pts',(5.33096558193683,4.81735099663587,2.90723060147415));
#19565=CARTESIAN_POINT('Ctrl Pts',(4.99079371715267,4.33896249921493,2.98534758100617));
#19566=CARTESIAN_POINT('Ctrl Pts',(4.95698752448753,3.74836627630877,3.06407671089558));
#19567=CARTESIAN_POINT('Ctrl Pts',(5.2447735927993,3.2263183390518,3.14340920265259));
#19568=CARTESIAN_POINT('Ctrl Pts',(5.77009659483826,2.935253839257,3.22333615530246));
#19569=CARTESIAN_POINT('Ctrl Pts',(6.37410700305503,2.96854764545913,3.3038436660997));
#19570=CARTESIAN_POINT('Ctrl Pts',(6.87126720532805,3.32056148618083,3.38491508906228));
#19571=CARTESIAN_POINT('Ctrl Pts',(7.10647606519176,3.8869115704884,3.46653020083125));
#19572=CARTESIAN_POINT('Ctrl Pts',(7.00364598168452,4.49544455922231,3.54866556866602));
#19573=CARTESIAN_POINT('Ctrl Pts',(6.59029031467595,4.95874770146656,3.63129490508721));
#19574=CARTESIAN_POINT('Ctrl Pts',(5.99050118891129,5.13204649144633,3.71438838994562));
#19575=CARTESIAN_POINT('Ctrl Pts',(5.3871831217877,4.95875602570457,3.7979148029937));
#19576=CARTESIAN_POINT('Ctrl Pts',(4.98248033378271,4.5061541351041,3.87872893188492));
#19577=CARTESIAN_POINT('Ctrl Pts',(4.86721670822546,3.93617018411993,3.9567542866616));
#19578=CARTESIAN_POINT('Ctrl Pts',(5.03201656034403,3.40093722969711,4.03191362348647));
#19579=CARTESIAN_POINT('Ctrl Pts',(5.4341155083194,3.00856657873451,4.10730454881205));
#19580=CARTESIAN_POINT('Ctrl Pts',(5.97619334481198,2.85552532694299,4.18289846038133));
#19581=CARTESIAN_POINT('Ctrl Pts',(6.52668855342533,2.98131870321029,4.25866237838478));
#19582=CARTESIAN_POINT('Ctrl Pts',(6.91525015578364,3.32433290152934,4.32823137789653));
#19583=CARTESIAN_POINT('Ctrl Pts',(7.10122540761753,3.75115514096909,4.39155786672224));
#19584=CARTESIAN_POINT('Ctrl Pts',(7.11704685769188,4.17012217382455,4.44859651091126));
#19585=CARTESIAN_POINT('Ctrl Pts',(6.97839397277603,4.56601865778953,4.50566782536761));
#19586=CARTESIAN_POINT('Ctrl Pts',(6.67448841900728,4.91976294635959,4.56909884830092));
#19587=CARTESIAN_POINT('Ctrl Pts',(6.20052248645988,5.13357708557862,4.63887978848427));
#19588=CARTESIAN_POINT('Ctrl Pts',(5.63509567281091,5.09095185636156,4.71498366372174));
#19589=CARTESIAN_POINT('Ctrl Pts',(5.19876269746781,4.80900916922666,4.78468292309207));
#19590=CARTESIAN_POINT('Ctrl Pts',(4.95194713053102,4.41489646436617,4.84798451555781));
#19591=CARTESIAN_POINT('Ctrl Pts',(4.84663163915403,3.86676853344418,4.92386073086651));
#19592=CARTESIAN_POINT('Ctrl Pts',(5.11372101102488,3.18474837462606,5.0184947367369));
#19593=CARTESIAN_POINT('Ctrl Pts',(5.90458358669118,2.80468201966577,5.13164482139767));
#19594=CARTESIAN_POINT('Ctrl Pts',(6.73806869810391,3.06284081116781,5.24427216882798));
#19595=CARTESIAN_POINT('Ctrl Pts',(7.17122830583924,3.81499585651111,5.35628592540322));
#19596=CARTESIAN_POINT('Ctrl Pts',(6.97836567750197,4.65554163951089,5.4675943780275));
#19597=CARTESIAN_POINT('Ctrl Pts',(6.26962123406518,5.13706960433728,5.57811808279645));
#19598=CARTESIAN_POINT('Ctrl Pts',(5.6171015280907,5.03711333283845,5.66341094659106));
#19599=CARTESIAN_POINT('Ctrl Pts',(5.26625724402755,4.76966136409525,5.72399491793109));
#19600=CARTESIAN_POINT('Ctrl Pts',(5.0466141008817,4.49503234360151,5.77232232410499));
#19601=CARTESIAN_POINT('Ctrl Pts',(4.91464587553303,4.06660447798485,5.83246573595406));
#19602=CARTESIAN_POINT('Ctrl Pts',(5.02121955424947,3.54300221950532,5.90419392967494));
#19603=CARTESIAN_POINT('Ctrl Pts',(5.36279729464331,3.13634388271878,5.97547169397601));
#19604=CARTESIAN_POINT('Ctrl Pts',(5.85400629104318,2.94418099963678,6.04628110835755));
#19605=CARTESIAN_POINT('Ctrl Pts',(6.33067382166986,3.00445097853177,6.11075992168625));
#19606=CARTESIAN_POINT('Ctrl Pts',(6.69244602053762,3.23270120290387,6.1690265414894));
#19607=CARTESIAN_POINT('Ctrl Pts',(6.99736200274051,3.64397358611959,6.23858290813363));
#19608=CARTESIAN_POINT('Ctrl Pts',(7.03741327745268,4.17541560408681,6.30760225841541));
#19609=CARTESIAN_POINT('Ctrl Pts',(6.79986566660976,4.6201895916107,6.37607276037605));
#19610=CARTESIAN_POINT('Ctrl Pts',(6.51581397770933,4.86495817257182,6.42715430300098));
#19611=CARTESIAN_POINT('Ctrl Pts',(6.16299958122418,4.9879746007512,6.47796790685504));
#19612=CARTESIAN_POINT('Ctrl Pts',(5.7298601965859,4.97194208493422,6.53693785301752));
#19613=CARTESIAN_POINT('Ctrl Pts',(5.28981334339032,4.7285935869624,6.60390272317146));
#19614=CARTESIAN_POINT('Ctrl Pts',(5.01861530795073,4.23654965453147,6.67865419687793));
#19615=CARTESIAN_POINT('Ctrl Pts',(5.04535351427297,3.77319789368563,6.740486484592));
#19616=CARTESIAN_POINT('Ctrl Pts',(5.21050707940139,3.45466912378663,6.78967190151324));
#19617=CARTESIAN_POINT('Ctrl Pts',(5.41498846216358,3.23821604795383,6.83051376083048));
#19618=CARTESIAN_POINT('Ctrl Pts',(5.70582623070768,3.08462360380577,6.87525912610462));
#19619=CARTESIAN_POINT('Ctrl Pts',(6.06055931995987,3.04484118040771,6.92384480353423));
#19620=CARTESIAN_POINT('Ctrl Pts',(6.4613286018102,3.1520453317179,6.98028088520478));
#19621=CARTESIAN_POINT('Ctrl Pts',(6.82054281279478,3.47314701577422,7.044453443696));
#19622=CARTESIAN_POINT('Ctrl Pts',(6.96928903457135,3.99139090417698,7.11621304917794));
#19623=CARTESIAN_POINT('Ctrl Pts',(6.82053867569686,4.50630577580192,7.18758304630547));
#19624=CARTESIAN_POINT('Ctrl Pts',(6.4225779203956,4.86150106821318,7.2585967677241));
#19625=CARTESIAN_POINT('Ctrl Pts',(5.89901648989417,4.95012788622332,7.32929565353266));
#19626=CARTESIAN_POINT('Ctrl Pts',(5.41042086398466,4.74746463183478,7.39972027350523));
#19627=CARTESIAN_POINT('Ctrl Pts',(5.10551074979547,4.31734756146974,7.46991401153098));
#19628=CARTESIAN_POINT('Ctrl Pts',(5.07619993383651,3.7923384190453,7.53992105125218));
#19629=CARTESIAN_POINT('Ctrl Pts',(5.33014973735899,3.33310630778287,7.60978689821025));
#19630=CARTESIAN_POINT('Ctrl Pts',(5.78885557715137,3.07967280968343,7.67955779837817));
#19631=CARTESIAN_POINT('Ctrl Pts',(6.31173203548677,3.10905948858246,7.74928060123239));
#19632=CARTESIAN_POINT('Ctrl Pts',(6.73885834106689,3.4120851493114,7.81900239890985));
#19633=CARTESIAN_POINT('Ctrl Pts',(6.93947166032782,3.89621327586067,7.88877032957341));
#19634=CARTESIAN_POINT('Ctrl Pts',(6.8517095108915,4.41356978513471,7.95863121731408));
#19635=CARTESIAN_POINT('Ctrl Pts',(6.5014540891724,4.80575205348109,8.02863146926931));
#19636=CARTESIAN_POINT('Ctrl Pts',(5.99497523815052,4.95190598589647,8.09881638421139));
#19637=CARTESIAN_POINT('Ctrl Pts',(5.48654071069358,4.80576306205798,8.16923084285141));
#19638=CARTESIAN_POINT('Ctrl Pts',(5.14584576047594,4.42467139458698,8.23729904032951));
#19639=CARTESIAN_POINT('Ctrl Pts',(5.04862865635048,3.94466948422526,8.30302425242081));
#19640=CARTESIAN_POINT('Ctrl Pts',(5.1876995521521,3.4935673709884,8.36639115082881));
#19641=CARTESIAN_POINT('Ctrl Pts',(5.49863720452088,3.18973076893938,8.42475458722929));
#19642=CARTESIAN_POINT('Ctrl Pts',(5.86851760288087,3.0604931366299,8.4780527344378));
#19643=CARTESIAN_POINT('Ctrl Pts',(6.22216787595036,3.07346286057778,8.52621481691567));
#19644=CARTESIAN_POINT('Ctrl Pts',(6.5480141776102,3.21557057599501,8.57457904463358));
#19645=CARTESIAN_POINT('Ctrl Pts',(6.80056307052306,3.4678858151066,8.62315683051673));
#19646=CARTESIAN_POINT('Ctrl Pts',(6.94413931041581,3.79655103609974,8.67195575349977));
#19647=CARTESIAN_POINT('Ctrl Pts',(6.95777663896381,4.1566166576575,8.72098348001793));
#19648=CARTESIAN_POINT('Ctrl Pts',(6.83835640468416,4.49842325083042,8.77024736714704));
#19649=CARTESIAN_POINT('Ctrl Pts',(6.60114870934877,4.77432525687952,8.81975397758997));
#19650=CARTESIAN_POINT('Ctrl Pts',(6.27792266149878,4.94535449549104,8.86950937083879));
#19651=CARTESIAN_POINT('Ctrl Pts',(5.91269004632584,4.9866810736209,8.91951878295217));
#19652=CARTESIAN_POINT('Ctrl Pts',(5.55577147754238,4.89123310443155,8.96978710902608));
#19653=CARTESIAN_POINT('Ctrl Pts',(5.25681276570615,4.67082116051935,9.02031786464434));
#19654=CARTESIAN_POINT('Ctrl Pts',(5.05804412704128,4.35480348104479,9.07111543725805));
#19655=CARTESIAN_POINT('Ctrl Pts',(4.98798705777152,3.98598291367431,9.12218002825493));
#19656=CARTESIAN_POINT('Ctrl Pts',(5.05811977792938,3.61529667809049,9.17351899333755));
#19657=CARTESIAN_POINT('Ctrl Pts',(5.28190831721568,3.25805572249925,9.23086036879321));
#19658=CARTESIAN_POINT('Ctrl Pts',(5.67891985984916,3.00111868286535,9.29432522451153));
#19659=CARTESIAN_POINT('Ctrl Pts',(6.19688560491034,2.9621595442335,9.36404551126668));
#19660=CARTESIAN_POINT('Ctrl Pts',(6.69384264119656,3.1855841651649,9.43716571018052));
#19661=CARTESIAN_POINT('Ctrl Pts',(7.02745653769267,3.65434324756386,9.51375564449963));
#19662=CARTESIAN_POINT('Ctrl Pts',(7.06178183126963,4.2554746146398,9.5938821811463));
#19663=CARTESIAN_POINT('Ctrl Pts',(6.76900853890664,4.78642987830011,9.67458399011126));
#19664=CARTESIAN_POINT('Ctrl Pts',(6.2348861539486,5.08229107067811,9.75584346418169));
#19665=CARTESIAN_POINT('Ctrl Pts',(5.62121277322736,5.04836986639924,9.83763914147065));
#19666=CARTESIAN_POINT('Ctrl Pts',(5.11650932635337,4.69091474437354,9.91994668477699));
#19667=CARTESIAN_POINT('Ctrl Pts',(4.87797688353407,4.11635214273989,10.0027386196848));
#19668=CARTESIAN_POINT('Ctrl Pts',(4.98229143524868,3.49959194392981,10.0859846604355));
#19669=CARTESIAN_POINT('Ctrl Pts',(5.40088841551943,3.03052905348384,10.1696518328908));
#19670=CARTESIAN_POINT('Ctrl Pts',(6.00767495654909,2.85530554851361,10.2537046813517));
#19671=CARTESIAN_POINT('Ctrl Pts',(6.61717928387298,3.0305340090082,10.3381054688078));
#19672=CARTESIAN_POINT('Ctrl Pts',(7.04154155207535,3.50493616550168,10.4228143856807));
#19673=CARTESIAN_POINT('Ctrl Pts',(7.14874926349887,4.13438019996447,10.5077898264163));
#19674=CARTESIAN_POINT('Ctrl Pts',(6.903950445343,4.72591482840965,10.5929885893347));
#19675=CARTESIAN_POINT('Ctrl Pts',(6.38082968565313,5.097277921466,10.6783661408612));
#19676=CARTESIAN_POINT('Ctrl Pts',(5.73930584472151,5.1334076879623,10.7638768930001));
#19677=CARTESIAN_POINT('Ctrl Pts',(5.1763348259103,4.82233123796325,10.8494744602056));
#19678=CARTESIAN_POINT('Ctrl Pts',(4.86504358341962,4.25912384558844,10.9351119396295));
#19679=CARTESIAN_POINT('Ctrl Pts',(4.90113867988794,3.616695945718,11.0207420968181));
#19680=CARTESIAN_POINT('Ctrl Pts',(5.27327395706588,3.09227155786067,11.1063179162021));
#19681=CARTESIAN_POINT('Ctrl Pts',(5.86665748296697,2.84661645816999,11.191792220633));
#19682=CARTESIAN_POINT('Ctrl Pts',(6.49864602437145,2.95402097485745,11.2771193627449));
#19683=CARTESIAN_POINT('Ctrl Pts',(6.97542925162609,3.38059696423684,11.3622524435191));
#19684=CARTESIAN_POINT('Ctrl Pts',(7.09288943197316,3.78884348331495,11.4188571787932));
#19685=CARTESIAN_POINT('Ctrl Pts',(7.09291698096067,3.9934841256345,11.4471081759746));
#19686=CARTESIAN_POINT('Ctrl Pts',(6.91041395631137,4.00974220039509,2.62934344456));
#19687=CARTESIAN_POINT('Ctrl Pts',(6.91039088332254,4.18113436374074,2.65300443127011));
#19688=CARTESIAN_POINT('Ctrl Pts',(6.81223276212051,4.52255345520787,2.70034331641334));
#19689=CARTESIAN_POINT('Ctrl Pts',(6.41194642259563,4.88120070727789,2.77187314650894));
#19690=CARTESIAN_POINT('Ctrl Pts',(5.87867709505731,4.97214216865051,2.84387604072737));
#19691=CARTESIAN_POINT('Ctrl Pts',(5.37495924775045,4.76411517635802,2.91641695294443));
#19692=CARTESIAN_POINT('Ctrl Pts',(5.05668129740466,4.31649040506209,2.98951203519711));
#19693=CARTESIAN_POINT('Ctrl Pts',(5.02502510535536,3.76378693926526,3.06319455885174));
#19694=CARTESIAN_POINT('Ctrl Pts',(5.29445839813617,3.27492491430021,3.13748525737848));
#19695=CARTESIAN_POINT('Ctrl Pts',(5.7867927450234,3.00204415093235,3.21240536311296));
#19696=CARTESIAN_POINT('Ctrl Pts',(6.35367476207417,3.03317811376964,3.28797059030528));
#19697=CARTESIAN_POINT('Ctrl Pts',(6.82113294013823,3.36398710098779,3.3641936508289));
#19698=CARTESIAN_POINT('Ctrl Pts',(7.04285181628566,3.89741148229682,3.44108302054775));
#19699=CARTESIAN_POINT('Ctrl Pts',(6.94595725577566,4.47200025222025,3.51864340064914));
#19700=CARTESIAN_POINT('Ctrl Pts',(6.55482461724248,4.91072870029518,3.59687544889804));
#19701=CARTESIAN_POINT('Ctrl Pts',(5.98546700894343,5.07548895052134,3.6757759027718));
#19702=CARTESIAN_POINT('Ctrl Pts',(5.410813879295,4.91071249002105,3.75533749097694));
#19703=CARTESIAN_POINT('Ctrl Pts',(5.02387704038526,4.47839131136037,3.83257833326237));
#19704=CARTESIAN_POINT('Ctrl Pts',(4.91313809632786,3.93191629171446,3.90740358805855));
#19705=CARTESIAN_POINT('Ctrl Pts',(5.07147125606051,3.41693922450177,3.97972471031443));
#19706=CARTESIAN_POINT('Ctrl Pts',(5.45948459805726,3.03797547396936,4.05251873428609));
#19707=CARTESIAN_POINT('Ctrl Pts',(5.98460263169843,2.889479086358,4.12576876881835));
#19708=CARTESIAN_POINT('Ctrl Pts',(6.51998892431244,3.01154612450741,4.19945421987059));
#19709=CARTESIAN_POINT('Ctrl Pts',(6.89944541092262,3.34622177075522,4.26738065081938));
#19710=CARTESIAN_POINT('Ctrl Pts',(7.08171822960832,3.76422693672321,4.32941579049949));
#19711=CARTESIAN_POINT('Ctrl Pts',(7.09737243151346,4.17579142315723,4.38545681087643));
#19712=CARTESIAN_POINT('Ctrl Pts',(6.96087151461153,4.5658912546307,4.44169554493835));
#19713=CARTESIAN_POINT('Ctrl Pts',(6.66065391126806,4.91555058236023,4.50439030579462));
#19714=CARTESIAN_POINT('Ctrl Pts',(6.1907350383217,5.12782606208152,4.57360248255073));
#19715=CARTESIAN_POINT('Ctrl Pts',(5.6277311318136,5.08567703703038,4.64938413671657));
#19716=CARTESIAN_POINT('Ctrl Pts',(5.19135680604461,4.80403271882307,4.71908080648419));
#19717=CARTESIAN_POINT('Ctrl Pts',(4.94362412438308,4.40869780521622,4.78259619492735));
#19718=CARTESIAN_POINT('Ctrl Pts',(4.83748052823326,3.85720781418724,4.85895645195229));
#19719=CARTESIAN_POINT('Ctrl Pts',(5.10669909946152,3.16750117053444,4.95464506809566));
#19720=CARTESIAN_POINT('Ctrl Pts',(5.91041143557091,2.78013675935754,5.06971853993261));
#19721=CARTESIAN_POINT('Ctrl Pts',(6.76309387143705,3.04322489315909,5.18492407896373));
#19722=CARTESIAN_POINT('Ctrl Pts',(7.20935006792413,3.81626935637355,5.30013664261463));
#19723=CARTESIAN_POINT('Ctrl Pts',(7.0108130147558,4.68549349365627,5.41523674764503));
#19724=CARTESIAN_POINT('Ctrl Pts',(6.27479660211849,5.18656709146719,5.53009928355427));
#19725=CARTESIAN_POINT('Ctrl Pts',(5.59341579180994,5.08278127978539,5.61916691846602));
#19726=CARTESIAN_POINT('Ctrl Pts',(5.22600755552765,4.80276063146936,5.68260544526989));
#19727=CARTESIAN_POINT('Ctrl Pts',(4.99568102716636,4.51482585519067,5.73328066698038));
#19728=CARTESIAN_POINT('Ctrl Pts',(4.85685941262204,4.06470665762287,5.79648169778678));
#19729=CARTESIAN_POINT('Ctrl Pts',(4.96895273785694,3.51311225847266,5.87204056226937));
#19730=CARTESIAN_POINT('Ctrl Pts',(5.32948706081087,3.08362490768829,5.94730430206206));
#19731=CARTESIAN_POINT('Ctrl Pts',(5.84918345972205,2.88016181192587,6.02222867343336));
#19732=CARTESIAN_POINT('Ctrl Pts',(6.35452293860915,2.94393317727708,6.09058427054729));
#19733=CARTESIAN_POINT('Ctrl Pts',(6.73862464213881,3.18621119370831,6.15244221152227));
#19734=CARTESIAN_POINT('Ctrl Pts',(7.06274421452183,3.62326913030874,6.22636742452222));
#19735=CARTESIAN_POINT('Ctrl Pts',(7.10554518164607,4.18887370461823,6.2998236824497));
#19736=CARTESIAN_POINT('Ctrl Pts',(6.85249430657903,4.66275908350551,6.37276822584886));
#19737=CARTESIAN_POINT('Ctrl Pts',(6.5497353495059,4.92367191327885,6.427214220678));
#19738=CARTESIAN_POINT('Ctrl Pts',(6.17354622005992,5.0548574765238,6.48139179108161));
#19739=CARTESIAN_POINT('Ctrl Pts',(5.71162272614039,5.03777059763326,6.54427708475726));
#19740=CARTESIAN_POINT('Ctrl Pts',(5.24233864535241,4.77825978354709,6.61568154310029));
#19741=CARTESIAN_POINT('Ctrl Pts',(4.95326379832803,4.25369877770726,6.69536188322357));
#19742=CARTESIAN_POINT('Ctrl Pts',(4.9818038280098,3.76014398076512,6.76121462096442));
#19743=CARTESIAN_POINT('Ctrl Pts',(5.15759473503968,3.42113765450785,6.81356035306079));
#19744=CARTESIAN_POINT('Ctrl Pts',(5.37509016478336,3.1909277463555,6.85699607265186));
#19745=CARTESIAN_POINT('Ctrl Pts',(5.68415420144532,3.02775093016466,6.9045368179429));
#19746=CARTESIAN_POINT('Ctrl Pts',(6.06065474879704,2.98556928880557,6.95609988254059));
#19747=CARTESIAN_POINT('Ctrl Pts',(6.48540963358703,3.0992501615105,7.01590966564209));
#19748=CARTESIAN_POINT('Ctrl Pts',(6.86525514523639,3.43902146271441,7.08377076212038));
#19749=CARTESIAN_POINT('Ctrl Pts',(7.02194275655083,3.98577375333824,7.1594543336964));
#19750=CARTESIAN_POINT('Ctrl Pts',(6.86526474012505,4.52718960725205,7.23449044610845));
#19751=CARTESIAN_POINT('Ctrl Pts',(6.44802096899966,4.89921223989767,7.30889435958139));
#19752=CARTESIAN_POINT('Ctrl Pts',(5.90137696830688,4.99143134985884,7.3826856212889));
#19753=CARTESIAN_POINT('Ctrl Pts',(5.3935204403864,4.78042083814242,7.45588715879427));
#19754=CARTESIAN_POINT('Ctrl Pts',(5.07819974972354,4.33501283869676,7.52852550298435));
#19755=CARTESIAN_POINT('Ctrl Pts',(5.04836966910811,3.79411731586998,7.60063046330751));
#19756=CARTESIAN_POINT('Ctrl Pts',(5.3090380544754,3.32352514962416,7.67223501391727));
#19757=CARTESIAN_POINT('Ctrl Pts',(5.77705219363671,3.0653997276032,7.74337509741105));
#19758=CARTESIAN_POINT('Ctrl Pts',(6.30747322592026,3.09561541382198,7.81408939563241));
#19759=CARTESIAN_POINT('Ctrl Pts',(6.73819282943324,3.40169434914954,7.88441910853963));
#19760=CARTESIAN_POINT('Ctrl Pts',(6.93910806394902,3.88763263418749,7.95440767991678));
#19761=CARTESIAN_POINT('Ctrl Pts',(6.85112713024168,4.4038038474583,8.0241006414166));
#19762=CARTESIAN_POINT('Ctrl Pts',(6.50326151996229,4.7926944191776,8.09354511221756));
#19763=CARTESIAN_POINT('Ctrl Pts',(6.00333540186104,4.93653882033147,8.16278997813517));
#19764=CARTESIAN_POINT('Ctrl Pts',(5.50441916176864,4.79271928260646,8.23188457022676));
#19765=CARTESIAN_POINT('Ctrl Pts',(5.17207445064451,4.42041718422104,8.29832531955615));
#19766=CARTESIAN_POINT('Ctrl Pts',(5.07788587706047,3.95400303163662,8.36216766357889));
#19767=CARTESIAN_POINT('Ctrl Pts',(5.21265715790399,3.51770078467468,8.42345990505972));
#19768=CARTESIAN_POINT('Ctrl Pts',(5.51233434006309,3.2251590091176,8.47967535154844));
#19769=CARTESIAN_POINT('Ctrl Pts',(5.86742948238684,3.10120558648341,8.5308308382066));
#19770=CARTESIAN_POINT('Ctrl Pts',(6.20594579383189,3.11370842761258,8.57692529727691));
#19771=CARTESIAN_POINT('Ctrl Pts',(6.51698026701549,3.24945320517786,8.62309340190623));
#19772=CARTESIAN_POINT('Ctrl Pts',(6.75739703043113,3.48976264907366,8.6693433903864));
#19773=CARTESIAN_POINT('Ctrl Pts',(6.89370889027547,3.80199715581543,8.71569298005573));
#19774=CARTESIAN_POINT('Ctrl Pts',(6.90655985977003,4.1432652519204,8.76215627878458));
#19775=CARTESIAN_POINT('Ctrl Pts',(6.79354285202102,4.46653335133218,8.80874733498412));
#19776=CARTESIAN_POINT('Ctrl Pts',(6.5695603815772,4.72695397581073,8.85547977713278));
#19777=CARTESIAN_POINT('Ctrl Pts',(6.26491749594757,4.88808364461752,8.90236695576895));
#19778=CARTESIAN_POINT('Ctrl Pts',(5.92123641980304,4.9269181534952,8.94942165494987));
#19779=CARTESIAN_POINT('Ctrl Pts',(5.5858502843238,4.83717950428668,8.99665654543328));
#19780=CARTESIAN_POINT('Ctrl Pts',(5.30526969819355,4.63026563478705,9.04408310168556));
#19781=CARTESIAN_POINT('Ctrl Pts',(5.11891531372185,4.33392015026218,9.09171390978302));
#19782=CARTESIAN_POINT('Ctrl Pts',(5.05330589123466,3.9883501365582,9.13955739856502));
#19783=CARTESIAN_POINT('Ctrl Pts',(5.11899493172307,3.6412513623554,9.18762957658963));
#19784=CARTESIAN_POINT('Ctrl Pts',(5.32847426937091,3.30689099803783,9.24130025707792));
#19785=CARTESIAN_POINT('Ctrl Pts',(5.69997317447753,3.06648203612493,9.30068647560233));
#19786=CARTESIAN_POINT('Ctrl Pts',(6.18464433636351,3.03002057055539,9.36592638537837));
#19787=CARTESIAN_POINT('Ctrl Pts',(6.64981640514089,3.2391315820987,9.4343725386264));
#19788=CARTESIAN_POINT('Ctrl Pts',(6.96234369156499,3.67816136171562,9.50611611783732));
#19789=CARTESIAN_POINT('Ctrl Pts',(6.99462295056451,4.24181543701733,9.58125450744829));
#19790=CARTESIAN_POINT('Ctrl Pts',(6.71981073272738,4.74045274816967,9.65704281024789));
#19791=CARTESIAN_POINT('Ctrl Pts',(6.21743521044141,5.01890229447707,9.73349236226831));
#19792=CARTESIAN_POINT('Ctrl Pts',(5.63891991598065,4.9871041225948,9.81061030522054));
#19793=CARTESIAN_POINT('Ctrl Pts',(5.16186682104324,4.64948394918386,9.88839996415766));
#19794=CARTESIAN_POINT('Ctrl Pts',(4.9356339179361,4.10514857215579,9.96686064525732));
#19795=CARTESIAN_POINT('Ctrl Pts',(5.03452093290359,3.518955270116,10.0459877096733));
#19796=CARTESIAN_POINT('Ctrl Pts',(5.43342184506395,3.07154769488501,10.1257725741091));
#19797=CARTESIAN_POINT('Ctrl Pts',(6.01387310894385,2.90361920550412,10.2062027693304));
#19798=CARTESIAN_POINT('Ctrl Pts',(6.59922913848389,3.07157463742995,10.2872620089041));
#19799=CARTESIAN_POINT('Ctrl Pts',(7.00853371667816,3.52863910059409,10.3689302828098));
#19800=CARTESIAN_POINT('Ctrl Pts',(7.11263621676139,4.13774647513387,10.4511839831483));
#19801=CARTESIAN_POINT('Ctrl Pts',(6.87508273089367,4.71273794439707,10.5339960578494));
#19802=CARTESIAN_POINT('Ctrl Pts',(6.36477112712681,5.07547594405445,10.617336091636));
#19803=CARTESIAN_POINT('Ctrl Pts',(5.73597718249919,5.11128123267146,10.7011706822485));
#19804=CARTESIAN_POINT('Ctrl Pts',(5.18151627774125,4.80536128072055,10.7854632253289));
#19805=CARTESIAN_POINT('Ctrl Pts',(4.87330818584072,4.24855973184745,10.8701750508535));
#19806=CARTESIAN_POINT('Ctrl Pts',(4.90876847724506,3.61030646882263,10.9552635490111));
#19807=CARTESIAN_POINT('Ctrl Pts',(5.27983677698369,3.08670458823981,11.0406871999814));
#19808=CARTESIAN_POINT('Ctrl Pts',(5.87458924075183,2.84003988052371,11.1263951356316));
#19809=CARTESIAN_POINT('Ctrl Pts',(6.51115887436203,2.94783391493837,11.2123513205601));
#19810=CARTESIAN_POINT('Ctrl Pts',(6.9937846298432,3.3790160528969,11.2984813503604));
#19811=CARTESIAN_POINT('Ctrl Pts',(7.11344785233266,3.79388082621453,11.3560322122809));
#19812=CARTESIAN_POINT('Ctrl Pts',(7.11347588125071,4.00208651046483,11.3847753697116));
#19813=CARTESIAN_POINT('Ctrl Pts',(6.88853591840586,3.99650689970452,2.72519413979724));
#19814=CARTESIAN_POINT('Ctrl Pts',(6.88851341699097,4.16365326312163,2.74826898643115));
#19815=CARTESIAN_POINT('Ctrl Pts',(6.79266132912078,4.49561543834634,2.79432441580812));
#19816=CARTESIAN_POINT('Ctrl Pts',(6.40608079986764,4.84117188888936,2.86333876459104));
#19817=CARTESIAN_POINT('Ctrl Pts',(5.89537064758869,4.92774941819879,2.93229843077413));
#19818=CARTESIAN_POINT('Ctrl Pts',(5.41672830057912,4.72953509189751,3.00126588273576));
#19819=CARTESIAN_POINT('Ctrl Pts',(5.1166250583807,4.306672709096,3.0702877604942));
#19820=CARTESIAN_POINT('Ctrl Pts',(5.08736771323111,3.78819012895638,3.13941747286813));
#19821=CARTESIAN_POINT('Ctrl Pts',(5.33896547323245,3.33253574183947,3.20870462329262));
#19822=CARTESIAN_POINT('Ctrl Pts',(5.79575192905363,3.0797864907763,3.2781993000075));
#19823=CARTESIAN_POINT('Ctrl Pts',(6.31891351953487,3.10885774055101,3.34794975500218));
#19824=CARTESIAN_POINT('Ctrl Pts',(6.74830379130066,3.41309068747734,3.41800297292553));
#19825=CARTESIAN_POINT('Ctrl Pts',(6.9510547607877,3.90154096365469,3.48840404180388));
#19826=CARTESIAN_POINT('Ctrl Pts',(6.86241953458854,4.42589831502308,3.55919606926937));
#19827=CARTESIAN_POINT('Ctrl Pts',(6.50623747712959,4.82517934530622,3.6304197748152));
#19828=CARTESIAN_POINT('Ctrl Pts',(5.98889285076722,4.97476706941445,3.70211342690322));
#19829=CARTESIAN_POINT('Ctrl Pts',(5.46747192638199,4.8251815280753,3.77431232631917));
#19830=CARTESIAN_POINT('Ctrl Pts',(5.11662658985994,4.43315301524721,3.84435526801514));
#19831=CARTESIAN_POINT('Ctrl Pts',(5.0162071016671,3.93768277376914,3.91219951548457));
#19832=CARTESIAN_POINT('Ctrl Pts',(5.15977522500822,3.47058203038587,3.97779639510337));
#19833=CARTESIAN_POINT('Ctrl Pts',(5.51194317996123,3.12652950334333,4.04387582993469));
#19834=CARTESIAN_POINT('Ctrl Pts',(5.98918621922857,2.99147246645262,4.11045074635524));
#19835=CARTESIAN_POINT('Ctrl Pts',(6.47663417367841,3.10248144007294,4.17753425939164));
#19836=CARTESIAN_POINT('Ctrl Pts',(6.82290650696304,3.40770249174057,4.23950079369268));
#19837=CARTESIAN_POINT('Ctrl Pts',(6.98963188577769,3.78984374605777,4.29621647725658));
#19838=CARTESIAN_POINT('Ctrl Pts',(7.00405510461931,4.16689870078161,4.34755696018617));
#19839=CARTESIAN_POINT('Ctrl Pts',(6.87879627909334,4.52513383179102,4.3991953454124));
#19840=CARTESIAN_POINT('Ctrl Pts',(6.60253522883494,4.84705653984927,4.45690236045491));
#19841=CARTESIAN_POINT('Ctrl Pts',(6.16873251221955,5.0432623691803,4.52080477312751));
#19842=CARTESIAN_POINT('Ctrl Pts',(5.64686447947036,5.00445557767878,4.59104407195184));
#19843=CARTESIAN_POINT('Ctrl Pts',(5.24057841000959,4.74254800820931,4.65590513107035));
#19844=CARTESIAN_POINT('Ctrl Pts',(5.00899522734369,4.37323225008896,4.71524515543419));
#19845=CARTESIAN_POINT('Ctrl Pts',(4.90930575929946,3.85626092864323,4.78683239775795));
#19846=CARTESIAN_POINT('Ctrl Pts',(5.16217234267391,3.20584850382231,4.87700824930854));
#19847=CARTESIAN_POINT('Ctrl Pts',(5.92497230789985,2.83677900383088,4.98629122769906));
#19848=CARTESIAN_POINT('Ctrl Pts',(6.74181256947623,3.08741194554306,5.09658083633684));
#19849=CARTESIAN_POINT('Ctrl Pts',(7.17390551165445,3.83314161511176,5.20780897590628));
#19850=CARTESIAN_POINT('Ctrl Pts',(6.9819580933047,4.68005707673005,5.31989205932659));
#19851=CARTESIAN_POINT('Ctrl Pts',(6.25953768149135,5.17368984108256,5.43274490177106));
#19852=CARTESIAN_POINT('Ctrl Pts',(5.58375279011301,5.07190606246186,5.52103398200387));
#19853=CARTESIAN_POINT('Ctrl Pts',(5.2171264186678,4.79260977215518,5.5843153809332));
#19854=CARTESIAN_POINT('Ctrl Pts',(4.98662050379357,4.50455297353126,5.63501958507542));
#19855=CARTESIAN_POINT('Ctrl Pts',(4.84672720555121,4.05225844509292,5.69852705507437));
#19856=CARTESIAN_POINT('Ctrl Pts',(4.95966976348219,3.49436670478253,5.77493252184398));
#19857=CARTESIAN_POINT('Ctrl Pts',(5.32608503302576,3.0571941642239,5.85147820369518));
#19858=CARTESIAN_POINT('Ctrl Pts',(5.8577786092087,2.84858806490979,5.92814817914561));
#19859=CARTESIAN_POINT('Ctrl Pts',(6.37799519612005,2.91385241516062,5.99849589652758));
#19860=CARTESIAN_POINT('Ctrl Pts',(6.77547364153904,3.16436890535246,6.06248319318287));
#19861=CARTESIAN_POINT('Ctrl Pts',(7.11240362358294,3.61827672062001,6.13928266561096));
#19862=CARTESIAN_POINT('Ctrl Pts',(7.15797797270208,4.20949068534465,6.21606342305039));
#19863=CARTESIAN_POINT('Ctrl Pts',(6.89201175633327,4.70809482040669,6.29277578692436));
#19864=CARTESIAN_POINT('Ctrl Pts',(6.5724187217174,4.98368655111803,6.35025944479518));
#19865=CARTESIAN_POINT('Ctrl Pts',(6.17373978783784,5.12287881823028,6.40767588785302));
#19866=CARTESIAN_POINT('Ctrl Pts',(5.6823406060203,5.10487059568676,6.47456829482958));
#19867=CARTESIAN_POINT('Ctrl Pts',(5.18072214992889,4.82794627066138,6.55085129832865));
#19868=CARTESIAN_POINT('Ctrl Pts',(4.86989576148384,4.26483639020975,6.6364092234611));
#19869=CARTESIAN_POINT('Ctrl Pts',(4.90037489921811,3.73231934687877,6.70744530149903));
#19870=CARTESIAN_POINT('Ctrl Pts',(5.09060477626466,3.36533950373994,6.76410150852154));
#19871=CARTESIAN_POINT('Ctrl Pts',(5.32647007599838,3.11562298111662,6.81120994313773));
#19872=CARTESIAN_POINT('Ctrl Pts',(5.66240586094145,2.93816076053336,6.86288601770773));
#19873=CARTESIAN_POINT('Ctrl Pts',(6.07267376915363,2.89210993004352,6.91907319999429));
#19874=CARTESIAN_POINT('Ctrl Pts',(6.53657749618968,3.016168195929,6.98439028889556));
#19875=CARTESIAN_POINT('Ctrl Pts',(6.95258373625134,3.38800637185586,7.05868183418768));
#19876=CARTESIAN_POINT('Ctrl Pts',(7.12475935034317,3.98808875937962,7.14175072442539));
#19877=CARTESIAN_POINT('Ctrl Pts',(6.95257123106385,4.58361106956866,7.22427606622913));
#19878=CARTESIAN_POINT('Ctrl Pts',(6.49303830168486,4.99347016775034,7.30623022342229));
#19879=CARTESIAN_POINT('Ctrl Pts',(5.89034148039216,5.09519412736382,7.38758739392877));
#19880=CARTESIAN_POINT('Ctrl Pts',(5.33019215632419,4.86245516950243,7.46832600555826));
#19881=CARTESIAN_POINT('Ctrl Pts',(4.98251724298352,4.37125724635345,7.54842784023342));
#19882=CARTESIAN_POINT('Ctrl Pts',(4.94974967352826,3.77526621848903,7.62787859492608));
#19883=CARTESIAN_POINT('Ctrl Pts',(5.23669328797984,3.25754942406365,7.70666776492358));
#19884=CARTESIAN_POINT('Ctrl Pts',(5.75070173993439,2.97428478802163,7.78478878417218));
#19885=CARTESIAN_POINT('Ctrl Pts',(6.33159360940416,3.00762384511478,7.86223904300809));
#19886=CARTESIAN_POINT('Ctrl Pts',(6.80161058800981,3.34199006094381,7.93901989429612));
#19887=CARTESIAN_POINT('Ctrl Pts',(7.01978160705851,3.87055260702782,8.01513669056237));
#19888=CARTESIAN_POINT('Ctrl Pts',(6.92415093523139,4.4293210351719,8.09059864737362));
#19889=CARTESIAN_POINT('Ctrl Pts',(6.54909128246045,4.84797549588681,8.16541903687084));
#19890=CARTESIAN_POINT('Ctrl Pts',(6.01337289669146,5.00163880577969,8.23961455650487));
#19891=CARTESIAN_POINT('Ctrl Pts',(5.48221378560674,4.84800085529194,8.31320646706303));
#19892=CARTESIAN_POINT('Ctrl Pts',(5.13096340100248,4.45377036243691,8.38351366750994));
#19893=CARTESIAN_POINT('Ctrl Pts',(5.0323627385332,3.96342516463837,8.45063523838859));
#19894=CARTESIAN_POINT('Ctrl Pts',(5.17348012374935,3.50789656631037,8.51465204594588));
#19895=CARTESIAN_POINT('Ctrl Pts',(5.48462531819063,3.20468646323622,8.5729767503835));
#19896=CARTESIAN_POINT('Ctrl Pts',(5.85082414469273,3.0770670717881,8.6257335694851));
#19897=CARTESIAN_POINT('Ctrl Pts',(6.19802868040939,3.09006779633478,8.67302093640832));
#19898=CARTESIAN_POINT('Ctrl Pts',(6.51524369375132,3.22870235157436,8.72012161242978));
#19899=CARTESIAN_POINT('Ctrl Pts',(6.75904035177302,3.47264584559122,8.76705528956744));
#19900=CARTESIAN_POINT('Ctrl Pts',(6.89641512498249,3.7877651061662,8.81383112604662));
#19901=CARTESIAN_POINT('Ctrl Pts',(6.90913118561134,4.13020988967364,8.8604625749268));
#19902=CARTESIAN_POINT('Ctrl Pts',(6.79618735088614,4.45272948408653,8.90696311627191));
#19903=CARTESIAN_POINT('Ctrl Pts',(6.57378623389393,4.71104075738766,8.95334670323705));
#19904=CARTESIAN_POINT('Ctrl Pts',(6.27305956286147,4.8699014145379,8.99962747923577));
#19905=CARTESIAN_POINT('Ctrl Pts',(5.9357221399501,4.90784517615673,9.04582006230268));
#19906=CARTESIAN_POINT('Ctrl Pts',(5.60836506362981,4.82007977229222,9.09193886304559));
#19907=CARTESIAN_POINT('Ctrl Pts',(5.33601985642346,4.61903031325887,9.13799945638055));
#19908=CARTESIAN_POINT('Ctrl Pts',(5.15614735317848,4.33269414268254,9.18401540712671));
#19909=CARTESIAN_POINT('Ctrl Pts',(5.09325308188048,4.00055596071841,9.23000522886462));
#19910=CARTESIAN_POINT('Ctrl Pts',(5.15620973600908,3.66868476868572,9.27597664931677));
#19911=CARTESIAN_POINT('Ctrl Pts',(5.35571636274036,3.35056367593898,9.32706303832943));
#19912=CARTESIAN_POINT('Ctrl Pts',(5.70751229844252,3.12327742081827,9.38328160753747));
#19913=CARTESIAN_POINT('Ctrl Pts',(6.16358069736592,3.08928682181092,9.44467557644274));
#19914=CARTESIAN_POINT('Ctrl Pts',(6.59876471880261,3.28526401983893,9.50873877884771));
#19915=CARTESIAN_POINT('Ctrl Pts',(6.88933460899203,3.69410126773656,9.57552448067617));
#19916=CARTESIAN_POINT('Ctrl Pts',(6.91885957284284,4.21597246912463,9.64510202690896));
#19917=CARTESIAN_POINT('Ctrl Pts',(6.66534460241342,4.6753100918803,9.71495149050467));
#19918=CARTESIAN_POINT('Ctrl Pts',(6.20418003654574,4.93059951255799,9.78511897981019));
#19919=CARTESIAN_POINT('Ctrl Pts',(5.67516373318628,4.90128602603705,9.85564916097365));
#19920=CARTESIAN_POINT('Ctrl Pts',(5.24030440189317,4.59329235978987,9.92658430072516));
#19921=CARTESIAN_POINT('Ctrl Pts',(5.03464208436496,4.09806935869481,9.99796437337559));
#19922=CARTESIAN_POINT('Ctrl Pts',(5.12454249776034,3.56575273707643,10.0698266715612));
#19923=CARTESIAN_POINT('Ctrl Pts',(5.48643447703374,3.15993632476991,10.1422056370457));
#19924=CARTESIAN_POINT('Ctrl Pts',(6.01271392287784,3.00768903052729,10.2151326458219));
#19925=CARTESIAN_POINT('Ctrl Pts',(6.54349763804324,3.15994780518182,10.2886358327811));
#19926=CARTESIAN_POINT('Ctrl Pts',(6.91494568619907,3.57461636346068,10.362739935582));
#19927=CARTESIAN_POINT('Ctrl Pts',(7.00964422215364,4.12795701399743,10.4374661110181));
#19928=CARTESIAN_POINT('Ctrl Pts',(6.79360471822111,4.65131590326631,10.5128318772436));
#19929=CARTESIAN_POINT('Ctrl Pts',(6.32823247077128,4.98236955691082,10.5888509146754));
#19930=CARTESIAN_POINT('Ctrl Pts',(5.75307679168745,5.01537468552453,10.6655331787411));
#19931=CARTESIAN_POINT('Ctrl Pts',(5.24410756609962,4.7348917526285,10.742884420018));
#19932=CARTESIAN_POINT('Ctrl Pts',(4.95992757920285,4.22219252722917,10.8209071127285));
#19933=CARTESIAN_POINT('Ctrl Pts',(4.99235186719618,3.63187243362919,10.8995983136656));
#19934=CARTESIAN_POINT('Ctrl Pts',(5.33674913990765,3.14520401194109,10.978954454041));
#19935=CARTESIAN_POINT('Ctrl Pts',(5.89179984276686,2.91453821379093,11.0589607383006));
#19936=CARTESIAN_POINT('Ctrl Pts',(6.48919734801473,3.01525134459007,11.1396150305874));
#19937=CARTESIAN_POINT('Ctrl Pts',(6.94487769083775,3.42171931985768,11.2208745171675));
#19938=CARTESIAN_POINT('Ctrl Pts',(7.05870005155304,3.815329029949,11.2754818828969));
#19939=CARTESIAN_POINT('Ctrl Pts',(7.05872671706659,4.01340701081049,11.302826893231));
#19940=CARTESIAN_POINT('Ctrl Pts',(6.95029262135111,3.98586592400863,2.8023339809504));
#19941=CARTESIAN_POINT('Ctrl Pts',(6.95026862138668,4.16414390317928,2.82694556653004));
#19942=CARTESIAN_POINT('Ctrl Pts',(6.84792718615896,4.5177844756354,2.87600736738179));
#19943=CARTESIAN_POINT('Ctrl Pts',(6.43856542568346,4.88296437357288,2.94901039334306));
#19944=CARTESIAN_POINT('Ctrl Pts',(5.9018694632682,4.97345421083968,3.02146390050822));
#19945=CARTESIAN_POINT('Ctrl Pts',(5.40282206296231,4.76616717188768,3.09339167774406));
#19946=CARTESIAN_POINT('Ctrl Pts',(5.09265327923777,4.32810410990818,3.16483096852571));
#19947=CARTESIAN_POINT('Ctrl Pts',(5.06321414551164,3.79557395318726,3.23581733974785));
#19948=CARTESIAN_POINT('Ctrl Pts',(5.32006997075252,3.33168210304646,3.30639105613246));
#19949=CARTESIAN_POINT('Ctrl Pts',(5.78189556541544,3.07685647218943,3.37659389527627));
#19950=CARTESIAN_POINT('Ctrl Pts',(6.306061875331,3.10660643356699,3.44647025580914));
#19951=CARTESIAN_POINT('Ctrl Pts',(6.73237009263218,3.40941104882764,3.51606622649372));
#19952=CARTESIAN_POINT('Ctrl Pts',(6.9316072436104,3.89098016790843,3.58542967826506));
#19953=CARTESIAN_POINT('Ctrl Pts',(6.84438820818325,4.40338817674375,3.6546097587502));
#19954=CARTESIAN_POINT('Ctrl Pts',(6.49860128520392,4.79014614756173,3.7236568258037));
#19955=CARTESIAN_POINT('Ctrl Pts',(6.00070838434377,4.93352949682256,3.79262169707247));
#19956=CARTESIAN_POINT('Ctrl Pts',(5.50293131088009,4.79016627090571,3.86155636785902));
#19957=CARTESIAN_POINT('Ctrl Pts',(5.17063680870318,4.41814039231168,3.92795749478015));
#19958=CARTESIAN_POINT('Ctrl Pts',(5.07636925998576,3.95125665644089,3.99187052042054));
#19959=CARTESIAN_POINT('Ctrl Pts',(5.21117483005849,3.51372127284347,4.05331922475323));
#19960=CARTESIAN_POINT('Ctrl Pts',(5.53960334069174,3.19327535333874,4.11489824654019));
#19961=CARTESIAN_POINT('Ctrl Pts',(5.9823373196834,3.06825891093373,4.17664317907259));
#19962=CARTESIAN_POINT('Ctrl Pts',(6.43241040339628,3.171013191632,4.23858678154593));
#19963=CARTESIAN_POINT('Ctrl Pts',(6.75077514309817,3.45189471835957,4.29557699148632));
#19964=CARTESIAN_POINT('Ctrl Pts',(6.90357262708646,3.8023490484242,4.34758089802266));
#19965=CARTESIAN_POINT('Ctrl Pts',(6.91669227102758,4.14729325868632,4.39454536832608));
#19966=CARTESIAN_POINT('Ctrl Pts',(6.80227826449375,4.47431115711779,4.4416842867902));
#19967=CARTESIAN_POINT('Ctrl Pts',(6.55047858520176,4.76762293520717,4.49426709814841));
#19968=CARTESIAN_POINT('Ctrl Pts',(6.15584183189205,4.94600137762016,4.55239112642174));
#19969=CARTESIAN_POINT('Ctrl Pts',(5.68189599016463,4.91067414241561,4.61618004824093));
#19970=CARTESIAN_POINT('Ctrl Pts',(5.31334944790297,4.67303293352455,4.67501869728126));
#19971=CARTESIAN_POINT('Ctrl Pts',(5.10338347611459,4.33816626959968,4.72882135277698));
#19972=CARTESIAN_POINT('Ctrl Pts',(5.01302782279375,3.86952242328442,4.79371606071519));
#19973=CARTESIAN_POINT('Ctrl Pts',(5.24221807036005,3.27983659742701,4.87546960685059));
#19974=CARTESIAN_POINT('Ctrl Pts',(5.93445578696586,2.94465187737126,4.97466218599338));
#19975=CARTESIAN_POINT('Ctrl Pts',(6.67754359068945,3.17225885927868,5.07498409546016));
#19976=CARTESIAN_POINT('Ctrl Pts',(7.07221058258075,3.85238211276754,5.17647139035252));
#19977=CARTESIAN_POINT('Ctrl Pts',(6.89701951458861,4.62825631875594,5.27914495771684));
#19978=CARTESIAN_POINT('Ctrl Pts',(6.23259905843267,5.0832096411637,5.383014538537));
#19979=CARTESIAN_POINT('Ctrl Pts',(5.60711153340288,4.98967355080173,5.46472964281215));
#19980=CARTESIAN_POINT('Ctrl Pts',(5.2663779085538,4.73018677183093,5.52353337130786));
#19981=CARTESIAN_POINT('Ctrl Pts',(5.05171364146542,4.46199084803395,5.5707490667026));
#19982=CARTESIAN_POINT('Ctrl Pts',(4.92078549467062,4.0395025260862,5.63009241759321));
#19983=CARTESIAN_POINT('Ctrl Pts',(5.02647905426851,3.51580809914182,5.70180650062497));
#19984=CARTESIAN_POINT('Ctrl Pts',(5.37182956432014,3.10326403527445,5.77401633992653));
#19985=CARTESIAN_POINT('Ctrl Pts',(5.87572839886343,2.90518654899726,5.84670063747711));
#19986=CARTESIAN_POINT('Ctrl Pts',(6.37154973362849,2.96705284831529,5.91375284847424));
#19987=CARTESIAN_POINT('Ctrl Pts',(6.75224572110308,3.20681178865771,5.97503021185853));
#19988=CARTESIAN_POINT('Ctrl Pts',(7.07638792235092,3.64307049823467,6.04888072578777));
#19989=CARTESIAN_POINT('Ctrl Pts',(7.12132260031561,4.21508352475279,6.12319600542698));
#19990=CARTESIAN_POINT('Ctrl Pts',(6.86248721959487,4.70093424719145,6.19792697815681));
#19991=CARTESIAN_POINT('Ctrl Pts',(6.54991569820719,4.9706696069471,6.2541726650809));
#19992=CARTESIAN_POINT('Ctrl Pts',(6.15818047323317,5.10763090774658,6.31060524208711));
#19993=CARTESIAN_POINT('Ctrl Pts',(5.67309911779094,5.09006207003428,6.37664509975054));
#19994=CARTESIAN_POINT('Ctrl Pts',(5.17486457479785,4.81560940559756,6.45239362911762));
#19995=CARTESIAN_POINT('Ctrl Pts',(4.86361942238087,4.25305527288563,6.53792585077325));
#19996=CARTESIAN_POINT('Ctrl Pts',(4.89379279366011,3.7170803326296,6.60943330857812));
#19997=CARTESIAN_POINT('Ctrl Pts',(5.08612427336279,3.34581493448056,6.66674534164118));
#19998=CARTESIAN_POINT('Ctrl Pts',(5.32544793519665,3.09232128730982,6.71456119953622));
#19999=CARTESIAN_POINT('Ctrl Pts',(5.66766652291053,2.9113478329744,6.76722272989925));
#20000=CARTESIAN_POINT('Ctrl Pts',(6.08754047418379,2.86404827015208,6.82473109672799));
#20001=CARTESIAN_POINT('Ctrl Pts',(6.56446533915124,2.99137086868677,6.89188059793245));
#20002=CARTESIAN_POINT('Ctrl Pts',(6.9948034795662,3.37532226913545,6.96868485606649));
#20003=CARTESIAN_POINT('Ctrl Pts',(7.17447589821626,3.99939255468548,7.05510703351458));
#20004=CARTESIAN_POINT('Ctrl Pts',(6.99478586305713,4.62290022027637,7.1415001950612));
#20005=CARTESIAN_POINT('Ctrl Pts',(6.51124973729689,5.05490208931216,7.22781058645099));
#20006=CARTESIAN_POINT('Ctrl Pts',(5.87300274454341,5.16315754515052,7.31398823594912));
#20007=CARTESIAN_POINT('Ctrl Pts',(5.27626245766403,4.9157518535826,7.39998244609693));
#20008=CARTESIAN_POINT('Ctrl Pts',(4.90367513413411,4.39016440467849,7.48574424609843));
#20009=CARTESIAN_POINT('Ctrl Pts',(4.86799015684862,3.74901012697494,7.57122574167028));
#20010=CARTESIAN_POINT('Ctrl Pts',(5.17774721687189,3.18930879840211,7.65638083635298));
#20011=CARTESIAN_POINT('Ctrl Pts',(5.73539172659811,2.88158319015515,7.74116527706526));
#20012=CARTESIAN_POINT('Ctrl Pts',(6.36818588209908,2.91757763006315,7.82553703910839));
#20013=CARTESIAN_POINT('Ctrl Pts',(6.88204837896223,3.28278988050203,7.90945652939063));
#20014=CARTESIAN_POINT('Ctrl Pts',(7.12139665456226,3.86203573124861,7.99288684375915));
#20015=CARTESIAN_POINT('Ctrl Pts',(7.01652149023538,4.47596056050852,8.07579394418247));
#20016=CARTESIAN_POINT('Ctrl Pts',(6.60380764727744,4.93686361595779,8.15814694002924));
#20017=CARTESIAN_POINT('Ctrl Pts',(6.01340669994955,5.1063137023791,8.23991814821641));
#20018=CARTESIAN_POINT('Ctrl Pts',(5.42754910994287,4.93690500888135,8.32108351621778));
#20019=CARTESIAN_POINT('Ctrl Pts',(5.04007369566793,4.50201262108148,8.39863925632172));
#20020=CARTESIAN_POINT('Ctrl Pts',(4.93137859155377,3.96129875447802,8.47264958788783));
#20021=CARTESIAN_POINT('Ctrl Pts',(5.08692636002921,3.45942866529189,8.54318005789076));
#20022=CARTESIAN_POINT('Ctrl Pts',(5.42934549869753,3.12585970665682,8.60735193538348));
#20023=CARTESIAN_POINT('Ctrl Pts',(5.83165822285851,2.98571811631052,8.66530492450804));
#20024=CARTESIAN_POINT('Ctrl Pts',(6.21246456474204,3.00003223598118,8.71716377919619));
#20025=CARTESIAN_POINT('Ctrl Pts',(6.55969646693978,3.15186453981375,8.76872368553389));
#20026=CARTESIAN_POINT('Ctrl Pts',(6.8259494531735,3.41838435941792,8.81998539901463));
#20027=CARTESIAN_POINT('Ctrl Pts',(6.9755642780092,3.76179602113988,8.8709503807213));
#20028=CARTESIAN_POINT('Ctrl Pts',(6.98928884168203,4.13394589808556,8.92162065781717));
#20029=CARTESIAN_POINT('Ctrl Pts',(6.86681407627787,4.48337006318172,8.97199922594141));
#20030=CARTESIAN_POINT('Ctrl Pts',(6.62652491520876,4.76228735386696,9.0220897436674));
#20031=CARTESIAN_POINT('Ctrl Pts',(6.30278876416356,4.93316832549157,9.07189671302883));
#20032=CARTESIAN_POINT('Ctrl Pts',(5.94102679899387,4.97373221571464,9.12142526742994));
#20033=CARTESIAN_POINT('Ctrl Pts',(5.59138868673641,4.87985437017635,9.17068149916784));
#20034=CARTESIAN_POINT('Ctrl Pts',(5.30176249967057,4.66587278516982,9.21967172890531));
#20035=CARTESIAN_POINT('Ctrl Pts',(5.11137406242519,4.36251784809578,9.26840406968075));
#20036=CARTESIAN_POINT('Ctrl Pts',(5.04521374956906,4.01229501739208,9.31688487199643));
#20037=CARTESIAN_POINT('Ctrl Pts',(5.11143815667451,3.66404729438246,9.36512665025428));
#20038=CARTESIAN_POINT('Ctrl Pts',(5.31994828225278,3.3319162252874,9.41846785264938));
#20039=CARTESIAN_POINT('Ctrl Pts',(5.68539334341808,3.09625451819029,9.47682673755812));
#20040=CARTESIAN_POINT('Ctrl Pts',(6.15565647977621,3.06162098730779,9.54012238468101));
#20041=CARTESIAN_POINT('Ctrl Pts',(6.60100163878465,3.26265755064533,9.60569449848809));
#20042=CARTESIAN_POINT('Ctrl Pts',(6.89570937301901,3.67833292911367,9.6735261620696));
#20043=CARTESIAN_POINT('Ctrl Pts',(6.92483105663458,4.20415079497554,9.74361163355922));
#20044=CARTESIAN_POINT('Ctrl Pts',(6.67099570698278,4.66278589979716,9.81338629730187));
#20045=CARTESIAN_POINT('Ctrl Pts',(6.21376195556722,4.91519459272152,9.88289707992095));
#20046=CARTESIAN_POINT('Ctrl Pts',(5.69394817961782,4.88578391502196,9.95219218161089));
#20047=CARTESIAN_POINT('Ctrl Pts',(5.2704284246474,4.58509660282537,10.0213211982662));
#20048=CARTESIAN_POINT('Ctrl Pts',(5.07208140876076,4.10599195241877,10.0903346798588));
#20049=CARTESIAN_POINT('Ctrl Pts',(5.15889590488797,3.59526417833319,10.1592839032291));
#20050=CARTESIAN_POINT('Ctrl Pts',(5.50402205104487,3.2090411194233,10.228220499924));
#20051=CARTESIAN_POINT('Ctrl Pts',(6.00199645879297,3.06550206122486,10.2971961924685));
#20052=CARTESIAN_POINT('Ctrl Pts',(6.50067778126696,3.20903914088455,10.36626247131));
#20053=CARTESIAN_POINT('Ctrl Pts',(6.84730300699068,3.59664724321552,10.4354703171584));
#20054=CARTESIAN_POINT('Ctrl Pts',(6.93486943208826,4.11067038305685,10.5048698349302));
#20055=CARTESIAN_POINT('Ctrl Pts',(6.73489012085044,4.59418295967456,10.5745100316563));
#20056=CARTESIAN_POINT('Ctrl Pts',(6.30657877272509,4.89848198644666,10.6444384740937));
#20057=CARTESIAN_POINT('Ctrl Pts',(5.77951424249628,4.92845041178851,10.7147010700453));
#20058=CARTESIAN_POINT('Ctrl Pts',(5.31478041770119,4.67207846115156,10.7853416371438));
#20059=CARTESIAN_POINT('Ctrl Pts',(5.05610819831086,4.20500636751179,10.8564020181706));
#20060=CARTESIAN_POINT('Ctrl Pts',(5.0857236524593,3.66847144880372,10.9279210600486));
#20061=CARTESIAN_POINT('Ctrl Pts',(5.39836096900337,3.22685123457935,10.9999360428456));
#20062=CARTESIAN_POINT('Ctrl Pts',(5.90166701382885,3.01775491662855,11.0724787922852));
#20063=CARTESIAN_POINT('Ctrl Pts',(6.44319411191715,3.10903218763481,11.1455837238297));
#20064=CARTESIAN_POINT('Ctrl Pts',(6.85640687171147,3.47760741146192,11.2192690183675));
#20065=CARTESIAN_POINT('Ctrl Pts',(6.95974821813124,3.83468369063596,11.2688070325982));
#20066=CARTESIAN_POINT('Ctrl Pts',(6.95977245031394,4.01468629256983,11.2936567053819));
#20067=CARTESIAN_POINT('Ctrl Pts',(7.04959553802912,3.98592257196897,2.80202047748269));
#20068=CARTESIAN_POINT('Ctrl Pts',(7.0495690992628,4.18231660611977,2.82913301600999));
#20069=CARTESIAN_POINT('Ctrl Pts',(6.93670763939659,4.57248778363104,2.88326745767727));
#20070=CARTESIAN_POINT('Ctrl Pts',(6.48513783957581,4.97524495721263,2.96379219618304));
#20071=CARTESIAN_POINT('Ctrl Pts',(5.89334453615466,5.07498515734521,3.04369199870337));
#20072=CARTESIAN_POINT('Ctrl Pts',(5.3436674177044,4.84653025539157,3.12292768885556));
#20073=CARTESIAN_POINT('Ctrl Pts',(5.00268894202627,4.364666605717,3.2015021172331));
#20074=CARTESIAN_POINT('Ctrl Pts',(4.97060199746087,3.78028520191834,3.27940497399593));
#20075=CARTESIAN_POINT('Ctrl Pts',(5.25189686376874,3.27280517974582,3.35663745551683));
#20076=CARTESIAN_POINT('Ctrl Pts',(5.75566324646624,2.99519266925544,3.43320128228222));
#20077=CARTESIAN_POINT('Ctrl Pts',(6.32494220199028,3.02785866798993,3.50910361898767));
#20078=CARTESIAN_POINT('Ctrl Pts',(6.78559902355489,3.35554698913419,3.58435484937817));
#20079=CARTESIAN_POINT('Ctrl Pts',(6.99948495517654,3.87366139696321,3.65896947413428));
#20080=CARTESIAN_POINT('Ctrl Pts',(6.9057443504678,4.42157190324475,3.73296568507402));
#20081=CARTESIAN_POINT('Ctrl Pts',(6.53784970235839,4.83229882165359,3.80636524986796));
#20082=CARTESIAN_POINT('Ctrl Pts',(6.0120185388268,4.9831728555397,3.8791937398877));
#20083=CARTESIAN_POINT('Ctrl Pts',(5.49030359434556,4.83232797125952,3.9514794730774));
#20084=CARTESIAN_POINT('Ctrl Pts',(5.14491551233214,4.44480770004393,4.02059711342777));
#20085=CARTESIAN_POINT('Ctrl Pts',(5.0479581811976,3.9623880425108,4.08663861071243));
#20086=CARTESIAN_POINT('Ctrl Pts',(5.18665328053576,3.51366989283078,4.14969046197642));
#20087=CARTESIAN_POINT('Ctrl Pts',(5.52144387908019,3.18760766277227,4.2124195271213));
#20088=CARTESIAN_POINT('Ctrl Pts',(5.96918476728892,3.06163542220108,4.27485533009919));
#20089=CARTESIAN_POINT('Ctrl Pts',(6.42075590052292,3.16517226550806,4.33702918560133));
#20090=CARTESIAN_POINT('Ctrl Pts',(6.73764131916391,3.44527816927544,4.39381653717447));
#20091=CARTESIAN_POINT('Ctrl Pts',(6.88868453992805,3.79220587970527,4.4452957229999));
#20092=CARTESIAN_POINT('Ctrl Pts',(6.9014239480865,4.13174739805484,4.49153188786438));
#20093=CARTESIAN_POINT('Ctrl Pts',(6.78926083467742,4.45182215831981,4.537686425972));
#20094=CARTESIAN_POINT('Ctrl Pts',(6.54392791119181,4.73730781199865,4.58889653940956));
#20095=CARTESIAN_POINT('Ctrl Pts',(6.16188835455284,4.90959837589481,4.64515385611942));
#20096=CARTESIAN_POINT('Ctrl Pts',(5.70642127297529,4.87526922755841,4.70646658352592));
#20097=CARTESIAN_POINT('Ctrl Pts',(5.35472035963564,4.64809143307424,4.76265838587514));
#20098=CARTESIAN_POINT('Ctrl Pts',(5.15549332398101,4.33007449213792,4.81375040542114));
#20099=CARTESIAN_POINT('Ctrl Pts',(5.07028857275984,3.88705211223204,4.87509303555694));
#20100=CARTESIAN_POINT('Ctrl Pts',(5.28634012787146,3.33363343332018,4.95188316018201));
#20101=CARTESIAN_POINT('Ctrl Pts',(5.93164782183758,3.0223131911079,5.04430473366233));
#20102=CARTESIAN_POINT('Ctrl Pts',(6.61875955095355,3.23368682312109,5.13712617207152));
#20103=CARTESIAN_POINT('Ctrl Pts',(6.98100189521977,3.8594139762258,5.23045666115443));
#20104=CARTESIAN_POINT('Ctrl Pts',(6.82012199070105,4.56911642578432,5.32440729336752));
#20105=CARTESIAN_POINT('Ctrl Pts',(6.21438174550616,4.98333168153799,5.41907564338409));
#20106=CARTESIAN_POINT('Ctrl Pts',(5.64601111551489,4.89810409433884,5.49334396077527));
#20107=CARTESIAN_POINT('Ctrl Pts',(5.33675238476666,4.66257985438181,5.54671921479505));
#20108=CARTESIAN_POINT('Ctrl Pts',(5.14200509570064,4.41925435453228,5.58955596074641));
#20109=CARTESIAN_POINT('Ctrl Pts',(5.02329884761106,4.03614199037101,5.6433706981261));
#20110=CARTESIAN_POINT('Ctrl Pts',(5.1191125849183,3.56137279247644,5.70838602410505));
#20111=CARTESIAN_POINT('Ctrl Pts',(5.43225089045909,3.18724975970799,5.77386738846131));
#20112=CARTESIAN_POINT('Ctrl Pts',(5.88948590428537,3.00745078575737,5.8398243456203));
#20113=CARTESIAN_POINT('Ctrl Pts',(6.33993918152939,3.06356712623787,5.90073865605301));
#20114=CARTESIAN_POINT('Ctrl Pts',(6.68630103774357,3.281643012517,5.9564827830694));
#20115=CARTESIAN_POINT('Ctrl Pts',(6.98164902707351,3.67901114045406,6.02376017437336));
#20116=CARTESIAN_POINT('Ctrl Pts',(7.02302073970407,4.20135333823992,6.09162172997393));
#20117=CARTESIAN_POINT('Ctrl Pts',(6.78602411743671,4.64650551718066,6.16007682324628));
#20118=CARTESIAN_POINT('Ctrl Pts',(6.49909070922357,4.89422004985391,6.21171564553496));
#20119=CARTESIAN_POINT('Ctrl Pts',(6.13857069981332,5.02037382723854,6.26365251588237));
#20120=CARTESIAN_POINT('Ctrl Pts',(5.69092255994263,5.0042823319112,6.32459305942612));
#20121=CARTESIAN_POINT('Ctrl Pts',(5.22937221718097,4.75041640031949,6.39473200066671));
#20122=CARTESIAN_POINT('Ctrl Pts',(4.93943560573875,4.2272480207064,6.47429954512901));
#20123=CARTESIAN_POINT('Ctrl Pts',(4.96729044189316,3.72610694101108,6.54114487313096));
#20124=CARTESIAN_POINT('Ctrl Pts',(5.14776765309921,3.37754925528953,6.59494075995518));
#20125=CARTESIAN_POINT('Ctrl Pts',(5.37298367506959,3.13891109087616,6.63994398732567));
#20126=CARTESIAN_POINT('Ctrl Pts',(5.69607229062316,2.96790283821101,6.68966571674888));
#20127=CARTESIAN_POINT('Ctrl Pts',(6.09406846289833,2.92292294668928,6.74417634428119));
#20128=CARTESIAN_POINT('Ctrl Pts',(6.54797103049369,3.04391143962956,6.80807461413231));
#20129=CARTESIAN_POINT('Ctrl Pts',(6.95985684136888,3.4107619087104,6.88151530993674));
#20130=CARTESIAN_POINT('Ctrl Pts',(7.13332472888623,4.01122017583434,6.96467649622193));
#20131=CARTESIAN_POINT('Ctrl Pts',(6.95982343278046,4.61531141611138,7.04834174242524));
#20132=CARTESIAN_POINT('Ctrl Pts',(6.48878339297744,5.03693983688589,7.13247718093113));
#20133=CARTESIAN_POINT('Ctrl Pts',(5.86245106661389,5.14378361000877,7.21704381765844));
#20134=CARTESIAN_POINT('Ctrl Pts',(5.27256413639821,4.89987938398564,7.30200117388622));
#20135=CARTESIAN_POINT('Ctrl Pts',(4.90139038498953,4.3773522928813,7.3873059879696));
#20136=CARTESIAN_POINT('Ctrl Pts',(4.86502821487562,3.73517169107109,7.47291316808673));
#20137=CARTESIAN_POINT('Ctrl Pts',(5.17687462738846,3.17041769901572,7.55877575548064));
#20138=CARTESIAN_POINT('Ctrl Pts',(5.74277715992316,2.85743325263498,7.64484530314035));
#20139=CARTESIAN_POINT('Ctrl Pts',(6.38963489855515,2.89361944545362,7.73107212119948));
#20140=CARTESIAN_POINT('Ctrl Pts',(6.9187191736916,3.26891722683287,7.81740561936278));
#20141=CARTESIAN_POINT('Ctrl Pts',(7.16713887971585,3.86858697286563,7.90379453112234));
#20142=CARTESIAN_POINT('Ctrl Pts',(7.05839689228429,4.50852957543109,7.99018731647296));
#20143=CARTESIAN_POINT('Ctrl Pts',(6.62601310199284,4.99222557577811,8.07653223837689));
#20144=CARTESIAN_POINT('Ctrl Pts',(6.00334857456791,5.17148530967006,8.16277821990696));
#20145=CARTESIAN_POINT('Ctrl Pts',(5.38165839885184,4.9922465523275,8.24887388737063));
#20146=CARTESIAN_POINT('Ctrl Pts',(4.96800443896283,4.52864882133443,8.33158917444569));
#20147=CARTESIAN_POINT('Ctrl Pts',(4.85117478658458,3.94914585502282,8.41090469888688));
#20148=CARTESIAN_POINT('Ctrl Pts',(5.01835098519788,3.4087989648184,8.48682393505967));
#20149=CARTESIAN_POINT('Ctrl Pts',(5.38826105600529,3.04810149166825,8.55617605853122));
#20150=CARTESIAN_POINT('Ctrl Pts',(5.82446178240406,2.89603606129518,8.61900857472436));
#20151=CARTESIAN_POINT('Ctrl Pts',(6.23844478670011,2.9115042535862,8.67538067701557));
#20152=CARTESIAN_POINT('Ctrl Pts',(6.61688532979205,3.07688853253289,8.7315669438026));
#20153=CARTESIAN_POINT('Ctrl Pts',(6.90773379958755,3.36791951130435,8.78755016886496));
#20154=CARTESIAN_POINT('Ctrl Pts',(7.07153121235227,3.74371362143827,8.84332189045714));
#20155=CARTESIAN_POINT('Ctrl Pts',(7.08663687068224,4.15171765258172,8.89887156867244));
#20156=CARTESIAN_POINT('Ctrl Pts',(6.95219592530982,4.53543180820108,8.95418929170758));
#20157=CARTESIAN_POINT('Ctrl Pts',(6.6880103580244,4.84214885063303,9.00926577760877));
#20158=CARTESIAN_POINT('Ctrl Pts',(6.33165270552102,5.03028395831446,9.06409237500585));
#20159=CARTESIAN_POINT('Ctrl Pts',(5.93307245554462,5.07499809321821,9.11866106189048));
#20160=CARTESIAN_POINT('Ctrl Pts',(5.54759924064695,4.97151165964518,9.17296457300614));
#20161=CARTESIAN_POINT('Ctrl Pts',(5.22816739524818,4.73551233569201,9.22699615481349));
#20162=CARTESIAN_POINT('Ctrl Pts',(5.01816475646119,4.40089573947751,9.28075018194062));
#20163=CARTESIAN_POINT('Ctrl Pts',(4.94521345392731,4.01463120053756,9.33422083258747));
#20164=CARTESIAN_POINT('Ctrl Pts',(5.01824316678122,3.63071258185625,9.3874050984931));
#20165=CARTESIAN_POINT('Ctrl Pts',(5.24799706943758,3.26481359843454,9.44617471319816));
#20166=CARTESIAN_POINT('Ctrl Pts',(5.6502251992854,3.00554549082188,9.51040219827145));
#20167=CARTESIAN_POINT('Ctrl Pts',(6.16686070362202,2.96762831361979,9.5799410017488));
#20168=CARTESIAN_POINT('Ctrl Pts',(6.65496938010503,3.18815865352936,9.65182585432177));
#20169=CARTESIAN_POINT('Ctrl Pts',(6.97688124136035,3.64266404253884,9.72597671203471));
#20170=CARTESIAN_POINT('Ctrl Pts',(7.00827068820807,4.2153313758698,9.80231317287426));
#20171=CARTESIAN_POINT('Ctrl Pts',(6.73267428113183,4.71252703931205,9.87799134108143));
#20172=CARTESIAN_POINT('Ctrl Pts',(6.23899646839629,4.98458622955827,9.95302302099409));
#20173=CARTESIAN_POINT('Ctrl Pts',(5.68099320199377,4.95256567160738,10.027423911631));
#20174=CARTESIAN_POINT('Ctrl Pts',(5.22927488560303,4.63126501449131,10.1012134002294));
#20175=CARTESIAN_POINT('Ctrl Pts',(5.01940525157708,4.12297974971796,10.1744145091191));
#20176=CARTESIAN_POINT('Ctrl Pts',(5.11138476437155,3.58510769121428,10.2470537440621));
#20177=CARTESIAN_POINT('Ctrl Pts',(5.47273837574136,3.18157531771205,10.3191609244022));
#20178=CARTESIAN_POINT('Ctrl Pts',(5.98977815820753,3.03315035815018,10.3907690213261));
#20179=CARTESIAN_POINT('Ctrl Pts',(6.50319759533062,3.1815542672455,10.4619139574862));
#20180=CARTESIAN_POINT('Ctrl Pts',(6.85686949607748,3.57795788637289,10.5326344118016));
#20181=CARTESIAN_POINT('Ctrl Pts',(6.94499243867947,4.09891704429121,10.6029715505245));
#20182=CARTESIAN_POINT('Ctrl Pts',(6.74346098168736,4.58456532043327,10.6729688187474));
#20183=CARTESIAN_POINT('Ctrl Pts',(6.31627019450132,4.887312142168,10.7426716956951));
#20184=CARTESIAN_POINT('Ctrl Pts',(5.795341673966,4.91631882842212,10.8121273603339));
#20185=CARTESIAN_POINT('Ctrl Pts',(5.34010223460903,4.66449596467932,10.8813845319597));
#20186=CARTESIAN_POINT('Ctrl Pts',(5.08910582152276,4.21006227233519,10.9504929286156));
#20187=CARTESIAN_POINT('Ctrl Pts',(5.11824740678368,3.69248318848022,11.0195036110717));
#20188=CARTESIAN_POINT('Ctrl Pts',(5.41803510645164,3.26995302498951,11.0884671692244));
#20189=CARTESIAN_POINT('Ctrl Pts',(5.89665777295442,3.07167464695276,11.1574368344658));
#20190=CARTESIAN_POINT('Ctrl Pts',(6.40783698205076,3.15826894639442,11.2264605725725));
#20191=CARTESIAN_POINT('Ctrl Pts',(6.79514811505036,3.50438353372458,11.2955976693271));
#20192=CARTESIAN_POINT('Ctrl Pts',(6.89129494882835,3.83722633847608,11.3417784389734));
#20193=CARTESIAN_POINT('Ctrl Pts',(6.89131751554605,4.00485745751464,11.3649202069907));
#20194=CARTESIAN_POINT('Ctrl Pts',(7.11181267012463,3.99652273239337,2.72529718128223));
#20195=CARTESIAN_POINT('Ctrl Pts',(7.11178468677333,4.20439034555461,2.75399366737857));
#20196=CARTESIAN_POINT('Ctrl Pts',(6.99229223216342,4.61848724239578,2.81144215490518));
#20197=CARTESIAN_POINT('Ctrl Pts',(6.51084510877054,5.04852489640089,2.89735482262377));
#20198=CARTESIAN_POINT('Ctrl Pts',(5.87630191856414,5.15592088469205,2.98303846056107));
#20199=CARTESIAN_POINT('Ctrl Pts',(5.28386722272041,4.91015879874544,3.06841711173038));
#20200=CARTESIAN_POINT('Ctrl Pts',(4.9145125012227,4.38888837216266,3.15345806443366));
#20201=CARTESIAN_POINT('Ctrl Pts',(4.87928389931365,3.75390688897146,3.23811208568559));
#20202=CARTESIAN_POINT('Ctrl Pts',(5.18576872246578,3.20031945302301,3.32234049131729));
#20203=CARTESIAN_POINT('Ctrl Pts',(5.73675947135142,2.89636870787145,3.40610340503253));
#20204=CARTESIAN_POINT('Ctrl Pts',(6.36124760601299,2.93197456969596,3.48936533645486));
#20205=CARTESIAN_POINT('Ctrl Pts',(6.86778482310151,3.29207952654758,3.57209303776967));
#20206=CARTESIAN_POINT('Ctrl Pts',(7.10344047238253,3.8625851317704,3.65425674031009));
#20207=CARTESIAN_POINT('Ctrl Pts',(7.00017622835295,4.46664939122879,3.73582982897195));
#20208=CARTESIAN_POINT('Ctrl Pts',(6.59438164089154,4.91973828380643,3.81678932294849));
#20209=CARTESIAN_POINT('Ctrl Pts',(6.01434996676503,5.08614779432233,3.8971156725437));
#20210=CARTESIAN_POINT('Ctrl Pts',(5.43923281895913,4.91979331284352,3.97679344121952));
#20211=CARTESIAN_POINT('Ctrl Pts',(5.05902725730369,4.49304297642434,4.05288364110645));
#20212=CARTESIAN_POINT('Ctrl Pts',(4.95257325831611,3.96276829797434,4.12546370000634));
#20213=CARTESIAN_POINT('Ctrl Pts',(5.10483091704482,3.47063897988742,4.19460857244748));
#20214=CARTESIAN_POINT('Ctrl Pts',(5.47121169123484,3.11405819360807,4.26322320045));
#20215=CARTESIAN_POINT('Ctrl Pts',(5.95960289303118,2.97684769455774,4.3313087925169));
#20216=CARTESIAN_POINT('Ctrl Pts',(6.45031424924818,3.08960839143403,4.39887090237078));
#20217=CARTESIAN_POINT('Ctrl Pts',(6.79316783996351,3.39296276675552,4.46032401438958));
#20218=CARTESIAN_POINT('Ctrl Pts',(6.95590913286132,3.76709016690528,4.51582256357046));
#20219=CARTESIAN_POINT('Ctrl Pts',(6.96947563984585,4.13190120659762,4.56548949965626));
#20220=CARTESIAN_POINT('Ctrl Pts',(6.84930227955056,4.4744430496678,4.61488140862749));
#20221=CARTESIAN_POINT('Ctrl Pts',(6.58764593315853,4.77868262767437,4.66946120942211));
#20222=CARTESIAN_POINT('Ctrl Pts',(6.18225551372277,4.9611503415574,4.72912558162728));
#20223=CARTESIAN_POINT('Ctrl Pts',(5.70201072840316,4.92457567772025,4.79377016122326));
#20224=CARTESIAN_POINT('Ctrl Pts',(5.33371017211244,4.68624272668883,4.85262925464343));
#20225=CARTESIAN_POINT('Ctrl Pts',(5.12631604517545,4.35485736180581,4.90584700293184));
#20226=CARTESIAN_POINT('Ctrl Pts',(5.03823119748178,3.89554988294405,4.96941983405228));
#20227=CARTESIAN_POINT('Ctrl Pts',(5.26153480425679,3.32684298684606,5.04835443670511));
#20228=CARTESIAN_POINT('Ctrl Pts',(5.91872114617452,3.01150181035348,5.14235135887236));
#20229=CARTESIAN_POINT('Ctrl Pts',(6.60960846454723,3.22564167844968,5.23571236345597));
#20230=CARTESIAN_POINT('Ctrl Pts',(6.9687422296195,3.84900858745817,5.32855016113735));
#20231=CARTESIAN_POINT('Ctrl Pts',(6.80897809494767,4.54707899531827,5.42097218274486));
#20232=CARTESIAN_POINT('Ctrl Pts',(6.2185221854142,4.94907192935034,5.51310245919284));
#20233=CARTESIAN_POINT('Ctrl Pts',(5.67121374043677,4.86595150720937,5.5846135144994));
#20234=CARTESIAN_POINT('Ctrl Pts',(5.37535400789112,4.64052470549437,5.63568594851014));
#20235=CARTESIAN_POINT('Ctrl Pts',(5.18962770820761,4.40837799391791,5.67654309787549));
#20236=CARTESIAN_POINT('Ctrl Pts',(5.07723172202838,4.04462781608614,5.72760987253886));
#20237=CARTESIAN_POINT('Ctrl Pts',(5.1679712265145,3.59672197447019,5.78895382949468));
#20238=CARTESIAN_POINT('Ctrl Pts',(5.46198384079215,3.24594656268194,5.85036986553849));
#20239=CARTESIAN_POINT('Ctrl Pts',(5.88878751737239,3.07843715833668,5.91191699354614));
#20240=CARTESIAN_POINT('Ctrl Pts',(6.30702680268281,3.130800218481,5.96847061746492));
#20241=CARTESIAN_POINT('Ctrl Pts',(6.62732725037718,3.33259493887353,6.02002492173982));
#20242=CARTESIAN_POINT('Ctrl Pts',(6.89953522861249,3.6991031536565,6.08205338958629));
#20243=CARTESIAN_POINT('Ctrl Pts',(6.93707330790287,4.17870591212063,6.14434527738535));
#20244=CARTESIAN_POINT('Ctrl Pts',(6.72016811142097,4.58585169655692,6.20696438244068));
#20245=CARTESIAN_POINT('Ctrl Pts',(6.45817664569874,4.81195395482581,6.25410374705552));
#20246=CARTESIAN_POINT('Ctrl Pts',(6.12962873730158,4.92684991317051,6.30142897812927));
#20247=CARTESIAN_POINT('Ctrl Pts',(5.72233475360488,4.91214713707122,6.35687397377257));
#20248=CARTESIAN_POINT('Ctrl Pts',(5.30311893072218,4.68142574318532,6.4205848471383));
#20249=CARTESIAN_POINT('Ctrl Pts',(5.04016290371371,4.20675760408258,6.49276867761505));
#20250=CARTESIAN_POINT('Ctrl Pts',(5.0654509590544,3.75242640036876,6.55336954181421));
#20251=CARTESIAN_POINT('Ctrl Pts',(5.22905797852052,3.43645099374466,6.60213700890933));
#20252=CARTESIAN_POINT('Ctrl Pts',(5.43324248086317,3.22009850678106,6.64293793377372));
#20253=CARTESIAN_POINT('Ctrl Pts',(5.72623728673697,3.06500752266559,6.68803041467216));
#20254=CARTESIAN_POINT('Ctrl Pts',(6.0873718502829,3.02417318346181,6.73749378609368));
#20255=CARTESIAN_POINT('Ctrl Pts',(6.49958056237668,3.13401391730095,6.79552400870097));
#20256=CARTESIAN_POINT('Ctrl Pts',(6.87420872741322,3.46752510001163,6.86231602845205));
#20257=CARTESIAN_POINT('Ctrl Pts',(7.03246380655118,4.01466143396108,6.9381074668043));
#20258=CARTESIAN_POINT('Ctrl Pts',(6.87415380765172,4.56667427800113,7.01456110403573));
#20259=CARTESIAN_POINT('Ctrl Pts',(6.44261059075647,4.95330475149549,7.09168397047356));
#20260=CARTESIAN_POINT('Ctrl Pts',(5.86656660182286,5.05187894759815,7.16947948898233));
#20261=CARTESIAN_POINT('Ctrl Pts',(5.32169990338654,4.82695809503764,7.24794693879057));
#20262=CARTESIAN_POINT('Ctrl Pts',(4.97712665602631,4.34252758715332,7.32708169022306));
#20263=CARTESIAN_POINT('Ctrl Pts',(4.94283169583294,3.74409201934878,7.40687513104107));
#20264=CARTESIAN_POINT('Ctrl Pts',(5.23454002534415,3.21489657129935,7.48731477307834));
#20265=CARTESIAN_POINT('Ctrl Pts',(5.7672320759956,2.9197426119313,7.56838428888876));
#20266=CARTESIAN_POINT('Ctrl Pts',(6.37987364666838,2.95351657370839,7.65006364226415));
#20267=CARTESIAN_POINT('Ctrl Pts',(6.88421899375099,3.31062599964522,7.73232917532269));
#20268=CARTESIAN_POINT('Ctrl Pts',(7.12283689664109,3.88521461663155,7.81515382444631));
#20269=CARTESIAN_POINT('Ctrl Pts',(7.01849989442465,4.50259033063837,7.89850710335461));
#20270=CARTESIAN_POINT('Ctrl Pts',(6.59915021057424,4.97257211814702,7.98235568954449));
#20271=CARTESIAN_POINT('Ctrl Pts',(5.99079694830932,5.14832315832535,8.06666276416388));
#20272=CARTESIAN_POINT('Ctrl Pts',(5.37898192660989,4.97255939586612,8.15139017469558));
#20273=CARTESIAN_POINT('Ctrl Pts',(4.96880293534666,4.51373060196947,8.23334231554345));
#20274=CARTESIAN_POINT('Ctrl Pts',(4.85189260237043,3.93609133882039,8.31243675137032));
#20275=CARTESIAN_POINT('Ctrl Pts',(5.01914830539027,3.39401212655114,8.38858983618502));
#20276=CARTESIAN_POINT('Ctrl Pts',(5.39213568611697,3.02978414283731,8.45858049946112));
#20277=CARTESIAN_POINT('Ctrl Pts',(5.83456068242697,2.87532762833332,8.52233051921372));
#20278=CARTESIAN_POINT('Ctrl Pts',(6.2563976504673,2.89091867238319,8.57978396734133));
#20279=CARTESIAN_POINT('Ctrl Pts',(6.64379204089303,3.06001729220897,8.6372938912653));
#20280=CARTESIAN_POINT('Ctrl Pts',(6.94291241285394,3.35908198542517,8.69485646707076));
#20281=CARTESIAN_POINT('Ctrl Pts',(7.11219375897664,3.74701895770555,8.75245114097456));
#20282=CARTESIAN_POINT('Ctrl Pts',(7.12802991342669,4.17008904416397,8.81006290988188));
#20283=CARTESIAN_POINT('Ctrl Pts',(6.98819439685561,4.56971599002978,8.86767639059384));
#20284=CARTESIAN_POINT('Ctrl Pts',(6.71207735115476,4.89054230347235,8.92527629676472));
#20285=CARTESIAN_POINT('Ctrl Pts',(6.33801804257999,5.08820852708785,8.98284725480005));
#20286=CARTESIAN_POINT('Ctrl Pts',(5.91791219418438,5.13549865056329,9.04037419115003));
#20287=CARTESIAN_POINT('Ctrl Pts',(5.50999677470214,5.02614912712557,9.09784167989352));
#20288=CARTESIAN_POINT('Ctrl Pts',(5.17064513125212,4.77562145632555,9.15523549031463));
#20289=CARTESIAN_POINT('Ctrl Pts',(4.94667637881517,4.4190272401054,9.21253926230186));
#20290=CARTESIAN_POINT('Ctrl Pts',(4.86850226651354,4.00588978606312,9.26974207914286));
#20291=CARTESIAN_POINT('Ctrl Pts',(4.94674979828523,3.59384604350928,9.32682158908026));
#20292=CARTESIAN_POINT('Ctrl Pts',(5.19398219286077,3.19983307636047,9.39010188193961));
#20293=CARTESIAN_POINT('Ctrl Pts',(5.62842891406782,2.91948832571542,9.45950185374663));
#20294=CARTESIAN_POINT('Ctrl Pts',(6.18870266339045,2.87811165294531,9.53491940251957));
#20295=CARTESIAN_POINT('Ctrl Pts',(6.71997102700817,3.11786770005593,9.61315040836019));
#20296=CARTESIAN_POINT('Ctrl Pts',(7.07166502030134,3.61392112245275,9.69411147936232));
#20297=CARTESIAN_POINT('Ctrl Pts',(7.10629841501347,4.24102436441314,9.77770801648046));
#20298=CARTESIAN_POINT('Ctrl Pts',(6.8039201214026,4.78697294048121,9.86079179520847));
#20299=CARTESIAN_POINT('Ctrl Pts',(6.26092047221784,5.08640170649856,9.94333064976283));
#20300=CARTESIAN_POINT('Ctrl Pts',(5.64615625799004,5.05124065078467,10.0252959694532));
#20301=CARTESIAN_POINT('Ctrl Pts',(5.14798795819423,4.69698307302897,10.1066623869624));
#20302=CARTESIAN_POINT('Ctrl Pts',(4.91645457617,4.13627479051779,10.1874081215893));
#20303=CARTESIAN_POINT('Ctrl Pts',(5.01793256528969,3.5430565390177,10.2675150298338));
#20304=CARTESIAN_POINT('Ctrl Pts',(5.41620966151829,3.09841671767496,10.3469687588456));
#20305=CARTESIAN_POINT('Ctrl Pts',(5.98521736545867,2.9352135316976,10.425758809164));
#20306=CARTESIAN_POINT('Ctrl Pts',(6.54900266284988,3.09836831360138,10.5038786074306));
#20307=CARTESIAN_POINT('Ctrl Pts',(6.93620171362726,3.53270289666941,10.5813255353004));
#20308=CARTESIAN_POINT('Ctrl Pts',(7.03212844521887,4.10149823693161,10.6581009683996));
#20309=CARTESIAN_POINT('Ctrl Pts',(6.81265030124579,4.62953048443375,10.7342102141382));
#20310=CARTESIAN_POINT('Ctrl Pts',(6.34990419138725,4.95701529899763,10.8096625970708));
#20311=CARTESIAN_POINT('Ctrl Pts',(5.78867040436841,4.98785046291451,10.8844711453126));
#20312=CARTESIAN_POINT('Ctrl Pts',(5.30115181038354,4.71765871139221,10.9586530713657));
#20313=CARTESIAN_POINT('Ctrl Pts',(5.03427591020065,4.23348651379917,11.0322284145427));
#20314=CARTESIAN_POINT('Ctrl Pts',(5.06560848410314,3.68591130814391,11.1052227432768));
#20315=CARTESIAN_POINT('Ctrl Pts',(5.38101430423995,3.24226419953413,11.1776606464299));
#20316=CARTESIAN_POINT('Ctrl Pts',(5.880425539423,3.03597565027725,11.2495797762185));
#20317=CARTESIAN_POINT('Ctrl Pts',(6.40940541410578,3.12614693210119,11.320998883741));
#20318=CARTESIAN_POINT('Ctrl Pts',(6.80671016386546,3.48207591472185,11.391988806191));
#20319=CARTESIAN_POINT('Ctrl Pts',(6.904197876148,3.82112270576356,11.4389948979343));
#20320=CARTESIAN_POINT('Ctrl Pts',(6.90422079703474,3.99138467936354,11.4624998600071));
#20321=CARTESIAN_POINT('Ctrl Pts',(7.08935433048845,4.00976795535994,2.62933137786601));
#20322=CARTESIAN_POINT('Ctrl Pts',(7.08932686336054,4.21380092684516,2.65749848499914));
#20323=CARTESIAN_POINT('Ctrl Pts',(6.97222248731657,4.62104874946912,2.71397012399248));
#20324=CARTESIAN_POINT('Ctrl Pts',(6.49589922960142,5.04740557699651,2.79904527326321));
#20325=CARTESIAN_POINT('Ctrl Pts',(5.86337876953338,5.15502662682281,2.88445395646036));
#20326=CARTESIAN_POINT('Ctrl Pts',(5.26845987859067,4.90888461943479,2.97015008062398));
#20327=CARTESIAN_POINT('Ctrl Pts',(4.89468286073338,4.3823824272392,3.05608638842908));
#20328=CARTESIAN_POINT('Ctrl Pts',(4.85824684039757,3.73630572363291,3.14221390254607));
#20329=CARTESIAN_POINT('Ctrl Pts',(5.1716759823261,3.16895431263743,3.22848265655362));
#20330=CARTESIAN_POINT('Ctrl Pts',(5.73951488913489,2.85504085505817,3.31484179770815));
#20331=CARTESIAN_POINT('Ctrl Pts',(6.38760587314015,2.89141605633462,3.4012399391865));
#20332=CARTESIAN_POINT('Ctrl Pts',(6.91689078349781,3.26700626473913,3.48762550541587));
#20333=CARTESIAN_POINT('Ctrl Pts',(7.16497694333469,3.86619302167825,3.57394696350454));
#20334=CARTESIAN_POINT('Ctrl Pts',(7.05635514580648,4.50465829681448,3.66015318410991));
#20335=CARTESIAN_POINT('Ctrl Pts',(6.62546144591164,4.98650451426083,3.74619367966986));
#20336=CARTESIAN_POINT('Ctrl Pts',(6.00586863628371,5.16474080304245,3.83201908797416));
#20337=CARTESIAN_POINT('Ctrl Pts',(5.3881890155353,4.98652307294238,3.91758099817887));
#20338=CARTESIAN_POINT('Ctrl Pts',(4.97772947734064,4.52637645614127,3.99967581713145));
#20339=CARTESIAN_POINT('Ctrl Pts',(4.86215903700014,3.95201587014982,4.07830191834474));
#20340=CARTESIAN_POINT('Ctrl Pts',(5.02745816897514,3.41698964677923,4.15347339544051));
#20341=CARTESIAN_POINT('Ctrl Pts',(5.42685607245378,3.02799004848427,4.22830474934372));
#20342=CARTESIAN_POINT('Ctrl Pts',(5.96089630415468,2.87777906722125,4.30276944214858));
#20343=CARTESIAN_POINT('Ctrl Pts',(6.498883490902,3.00124378734206,4.3768415412266));
#20344=CARTESIAN_POINT('Ctrl Pts',(6.87559304456626,3.33442659112351,4.44436385892624));
#20345=CARTESIAN_POINT('Ctrl Pts',(7.05466837051393,3.74599838952216,4.50542711365477));
#20346=CARTESIAN_POINT('Ctrl Pts',(7.0696349027974,4.14774221788009,4.56013064700762));
#20347=CARTESIAN_POINT('Ctrl Pts',(6.93721352970015,4.5252554236123,4.61457214688294));
#20348=CARTESIAN_POINT('Ctrl Pts',(6.64870709702653,4.86073716900179,4.67476505846687));
#20349=CARTESIAN_POINT('Ctrl Pts',(6.20157167497753,5.06199839012352,4.74058479308716));
#20350=CARTESIAN_POINT('Ctrl Pts',(5.67194776490379,5.02164353040941,4.81188340787891));
#20351=CARTESIAN_POINT('Ctrl Pts',(5.26602157976127,4.75890044535489,4.87677636521827));
#20352=CARTESIAN_POINT('Ctrl Pts',(5.03768164384035,4.39397997563631,4.93538709414076));
#20353=CARTESIAN_POINT('Ctrl Pts',(4.94084027807397,3.88872668946754,5.00532561214801));
#20354=CARTESIAN_POINT('Ctrl Pts',(5.18635472219651,3.26450838263861,5.09201744883042));
#20355=CARTESIAN_POINT('Ctrl Pts',(5.90539913314412,2.9202105403707,5.19484754170443));
#20356=CARTESIAN_POINT('Ctrl Pts',(6.65711372555407,3.15403622799657,5.29649452650138));
#20357=CARTESIAN_POINT('Ctrl Pts',(7.04488820377841,3.82898969542974,5.39697458995052));
#20358=CARTESIAN_POINT('Ctrl Pts',(6.87215114063041,4.57889997706907,5.49632422913287));
#20359=CARTESIAN_POINT('Ctrl Pts',(6.24191793133484,5.00652110364668,5.59458304482695));
#20360=CARTESIAN_POINT('Ctrl Pts',(5.66351128855155,4.91769964682495,5.67021033793647));
#20361=CARTESIAN_POINT('Ctrl Pts',(5.35282932082097,4.68086189098653,5.72386333549739));
#20362=CARTESIAN_POINT('Ctrl Pts',(5.15839756524628,4.43774535650645,5.76664581513995));
#20363=CARTESIAN_POINT('Ctrl Pts',(5.04161323177532,4.05859515840377,5.81987839248399));
#20364=CARTESIAN_POINT('Ctrl Pts',(5.13590711786686,3.59516217764757,5.88336509719667));
#20365=CARTESIAN_POINT('Ctrl Pts',(5.43840686123041,3.23491925336827,5.94650403845761));
#20366=CARTESIAN_POINT('Ctrl Pts',(5.87402874651677,3.06439434962665,6.00930738120382));
#20367=CARTESIAN_POINT('Ctrl Pts',(6.29763282423888,3.11782006164934,6.06660731821252));
#20368=CARTESIAN_POINT('Ctrl Pts',(6.61987707815288,3.32104408260551,6.11849992137742));
#20369=CARTESIAN_POINT('Ctrl Pts',(6.89212340909391,3.68804846399038,6.18058610286788));
#20370=CARTESIAN_POINT('Ctrl Pts',(6.92849012913488,4.16419527438217,6.24242788479418));
#20371=CARTESIAN_POINT('Ctrl Pts',(6.71476440569141,4.56477929198679,6.30407569392624));
#20372=CARTESIAN_POINT('Ctrl Pts',(6.45817356746196,4.78602937621426,6.35022990420567));
#20373=CARTESIAN_POINT('Ctrl Pts',(6.13819352709224,4.89774520806743,6.39631813497738));
#20374=CARTESIAN_POINT('Ctrl Pts',(5.74367658479674,4.88331063715809,6.4500272795765));
#20375=CARTESIAN_POINT('Ctrl Pts',(5.34043473367568,4.66083857309541,6.51135079611151));
#20376=CARTESIAN_POINT('Ctrl Pts',(5.08972251749124,4.20716379117729,6.58030851727006));
#20377=CARTESIAN_POINT('Ctrl Pts',(5.11409780711009,3.77627756908702,6.63779196306467));
#20378=CARTESIAN_POINT('Ctrl Pts',(5.26855297760062,3.47814452242061,6.6838142751157));
#20379=CARTESIAN_POINT('Ctrl Pts',(5.46065965467812,3.27467109759302,6.72219367629874));
#20380=CARTESIAN_POINT('Ctrl Pts',(5.73530920658978,3.12942231351325,6.76445528686445));
#20381=CARTESIAN_POINT('Ctrl Pts',(6.07243948189482,3.09141890367305,6.81062897902484));
#20382=CARTESIAN_POINT('Ctrl Pts',(6.45577255332208,3.19370606878804,6.86459737973638));
#20383=CARTESIAN_POINT('Ctrl Pts',(6.80245632541254,3.50275472411468,6.92643953978416));
#20384=CARTESIAN_POINT('Ctrl Pts',(6.94799187214705,4.00707810157704,6.99628444477559));
#20385=CARTESIAN_POINT('Ctrl Pts',(6.80243463304903,4.51362937231149,7.06644698250257));
#20386=CARTESIAN_POINT('Ctrl Pts',(6.40761680157126,4.86704233480136,7.13697211191855));
#20387=CARTESIAN_POINT('Ctrl Pts',(5.88232251234982,4.95673954752656,7.2079018942272));
#20388=CARTESIAN_POINT('Ctrl Pts',(5.38670220439379,4.75199108710649,7.27927635011301));
#20389=CARTESIAN_POINT('Ctrl Pts',(5.07385848731881,4.311996570288,7.35113272577799));
#20390=CARTESIAN_POINT('Ctrl Pts',(5.04280233204593,3.76912795832174,7.42350548003733));
#20391=CARTESIAN_POINT('Ctrl Pts',(5.30729570140107,3.28932314010225,7.49642597611492));
#20392=CARTESIAN_POINT('Ctrl Pts',(5.79029685260329,3.02166150968425,7.56992236804696));
#20393=CARTESIAN_POINT('Ctrl Pts',(6.34617932999724,3.05222693602592,7.64401937762537));
#20394=CARTESIAN_POINT('Ctrl Pts',(6.80442436050835,3.37654354073427,7.718738186782));
#20395=CARTESIAN_POINT('Ctrl Pts',(7.0217323472939,3.89938565329031,7.79409624897815));
#20396=CARTESIAN_POINT('Ctrl Pts',(6.92676983345605,4.46254487713906,7.87010732284795));
#20397=CARTESIAN_POINT('Ctrl Pts',(6.54339548688279,4.89258459447592,7.94678107889299));
#20398=CARTESIAN_POINT('Ctrl Pts',(5.98523957875296,5.05413538621001,8.02412370189236));
#20399=CARTESIAN_POINT('Ctrl Pts',(5.42166576321615,4.89257860872644,8.10213637984392));
#20400=CARTESIAN_POINT('Ctrl Pts',(5.04208531888007,4.46849204652117,8.1779043724297));
#20401=CARTESIAN_POINT('Ctrl Pts',(4.93322033775504,3.93210456253714,8.25133605036051));
#20402=CARTESIAN_POINT('Ctrl Pts',(5.08894992358947,3.42641889652029,8.32235393730101));
#20403=CARTESIAN_POINT('Ctrl Pts',(5.43819988286549,3.08496270726174,8.3879176883461));
#20404=CARTESIAN_POINT('Ctrl Pts',(5.85439720026083,2.93950036803367,8.44788098607834));
#20405=CARTESIAN_POINT('Ctrl Pts',(6.25273505159805,2.95408037327976,8.50212064403883));
#20406=CARTESIAN_POINT('Ctrl Pts',(6.62002653788648,3.11424812103136,8.55663149134766));
#20407=CARTESIAN_POINT('Ctrl Pts',(6.90478701925602,3.39874133408262,8.61139845473666));
#20408=CARTESIAN_POINT('Ctrl Pts',(7.06667132637044,3.76934455991646,8.66641744103278));
#20409=CARTESIAN_POINT('Ctrl Pts',(7.08202020427562,4.17523803377879,8.72167975629805));
#20410=CARTESIAN_POINT('Ctrl Pts',(6.94744505752561,4.56031046139421,8.77717629140723));
#20411=CARTESIAN_POINT('Ctrl Pts',(6.68040413477401,4.87083756629178,8.83289726235809));
#20412=CARTESIAN_POINT('Ctrl Pts',(6.31698023363933,5.06306852888535,8.88883235968104));
#20413=CARTESIAN_POINT('Ctrl Pts',(5.90695649456619,5.10939104643414,8.94497057613671));
#20414=CARTESIAN_POINT('Ctrl Pts',(5.50700065253343,5.00234857682117,9.00130066835425));
#20415=CARTESIAN_POINT('Ctrl Pts',(5.17271431399361,4.75577353964803,9.05781022196116));
#20416=CARTESIAN_POINT('Ctrl Pts',(4.9510179457879,4.40311243255541,9.11448783483843));
#20417=CARTESIAN_POINT('Ctrl Pts',(4.87316516980905,3.99261893252283,9.17131834442002));
#20418=CARTESIAN_POINT('Ctrl Pts',(4.9511114040548,3.58126083564377,9.22829363176974));
#20419=CARTESIAN_POINT('Ctrl Pts',(5.19884658438153,3.18607396297299,9.29173818490542));
#20420=CARTESIAN_POINT('Ctrl Pts',(5.63659194270646,2.90314131258883,9.36168994453439));
#20421=CARTESIAN_POINT('Ctrl Pts',(6.20478195247466,2.86076221415241,9.43817021297446));
#20422=CARTESIAN_POINT('Ctrl Pts',(6.74696264486986,3.1049657067049,9.51797393250518));
#20423=CARTESIAN_POINT('Ctrl Pts',(7.10847634266124,3.61390080934243,9.60108201071482));
#20424=CARTESIAN_POINT('Ctrl Pts',(7.14484568778978,4.26189538676859,9.68745983808889));
#20425=CARTESIAN_POINT('Ctrl Pts',(6.83086847979655,4.82994556052449,9.77385907953142));
#20426=CARTESIAN_POINT('Ctrl Pts',(6.26290560133959,5.14376668795179,9.86022824454772));
#20427=CARTESIAN_POINT('Ctrl Pts',(5.61567071701958,5.10727846960762,9.94651578749562));
#20428=CARTESIAN_POINT('Ctrl Pts',(5.08788422817577,4.73257952185281,10.0326707962013));
#20429=CARTESIAN_POINT('Ctrl Pts',(4.84092239529325,4.13576460899181,10.1186430740689));
#20430=CARTESIAN_POINT('Ctrl Pts',(4.94909058655262,3.50076872538124,10.204383526189));
#20431=CARTESIAN_POINT('Ctrl Pts',(5.37714970392394,3.02225388968236,10.28984443812));
#20432=CARTESIAN_POINT('Ctrl Pts',(5.99183811975877,2.84554982415397,10.3749797497847));
#20433=CARTESIAN_POINT('Ctrl Pts',(6.60363354102406,3.0222373440814,10.4597453269029));
#20434=CARTESIAN_POINT('Ctrl Pts',(7.02555360958883,3.49505624895605,10.5440992034139));
#20435=CARTESIAN_POINT('Ctrl Pts',(7.13063773339451,4.11653821456178,10.6280018838759));
#20436=CARTESIAN_POINT('Ctrl Pts',(6.89033336017905,4.69526271422283,10.711416501209));
#20437=CARTESIAN_POINT('Ctrl Pts',(6.38213884592012,5.05513174920232,10.7943091108394));
#20438=CARTESIAN_POINT('Ctrl Pts',(5.76451938509553,5.0891965723836,10.876648761637));
#20439=CARTESIAN_POINT('Ctrl Pts',(5.22726652981424,4.79153165150449,10.9584079729608));
#20440=CARTESIAN_POINT('Ctrl Pts',(4.93293862223068,4.25760702694337,11.0395622174635));
#20441=CARTESIAN_POINT('Ctrl Pts',(4.96752800826392,3.65362765488133,11.1200915355985));
#20442=CARTESIAN_POINT('Ctrl Pts',(5.31535928228549,3.1645184205444,11.199977394954));
#20443=CARTESIAN_POINT('Ctrl Pts',(5.86551291199122,2.93739523900251,11.2792100321066));
#20444=CARTESIAN_POINT('Ctrl Pts',(6.44725074043973,3.03673721882636,11.3577722921244));
#20445=CARTESIAN_POINT('Ctrl Pts',(6.88309362092661,3.42739799729367,11.4356761752053));
#20446=CARTESIAN_POINT('Ctrl Pts',(6.98969439584974,3.79852728114815,11.4871433778357));
#20447=CARTESIAN_POINT('Ctrl Pts',(6.98971942206308,3.98442813763357,11.5128073149357));
#20448=CARTESIAN_POINT('Ctrl Pts',(7.02991808875681,4.01367950132643,2.60093950625072));
#20449=CARTESIAN_POINT('Ctrl Pts',(7.02989207675763,4.2069033980654,2.62761440178603));
#20450=CARTESIAN_POINT('Ctrl Pts',(6.91906228277925,4.59266109443473,2.68110100393894));
#20451=CARTESIAN_POINT('Ctrl Pts',(6.46673327264386,4.99790650328683,2.76192471741077));
#20452=CARTESIAN_POINT('Ctrl Pts',(5.86413112095171,5.10068618268087,2.84329382346269));
#20453=CARTESIAN_POINT('Ctrl Pts',(5.29540647873442,4.86571365741625,2.92519940248184));
#20454=CARTESIAN_POINT('Ctrl Pts',(4.93668483059122,4.36097545535027,3.00761016390175));
#20455=CARTESIAN_POINT('Ctrl Pts',(4.9012748009943,3.7391829555439,3.09050047048975));
#20456=CARTESIAN_POINT('Ctrl Pts',(5.20375531414926,3.19090833877407,3.17383809803486));
#20457=CARTESIAN_POINT('Ctrl Pts',(5.75430443912642,2.88613009498686,3.25758993339851));
#20458=CARTESIAN_POINT('Ctrl Pts',(6.38545139705114,2.92117220627119,3.3417196729076));
#20459=CARTESIAN_POINT('Ctrl Pts',(6.90327506386492,3.28814937452449,3.42618914575835));
#20460=CARTESIAN_POINT('Ctrl Pts',(7.14729913444027,3.87647832619913,3.51095806950405));
#20461=CARTESIAN_POINT('Ctrl Pts',(7.0405517643525,4.50636423470096,3.59598432294754));
#20462=CARTESIAN_POINT('Ctrl Pts',(6.6139053462151,4.98408502788234,3.68122453242074));
#20463=CARTESIAN_POINT('Ctrl Pts',(5.99731919977364,5.16189360299918,3.76663340605859));
#20464=CARTESIAN_POINT('Ctrl Pts',(5.3796093434696,4.98411146303029,3.85216606290971));
#20465=CARTESIAN_POINT('Ctrl Pts',(4.96703346331831,4.52220317024434,3.9346029099679));
#20466=CARTESIAN_POINT('Ctrl Pts',(4.85014913796247,3.94288660972667,4.01389923751922));
#20467=CARTESIAN_POINT('Ctrl Pts',(5.01727777754471,3.40093747399747,4.09001126566938));
#20468=CARTESIAN_POINT('Ctrl Pts',(5.42319114007935,3.00520029144226,4.16608362665331));
#20469=CARTESIAN_POINT('Ctrl Pts',(5.96826825075608,2.85157652510321,4.24208401642723));
#20470=CARTESIAN_POINT('Ctrl Pts',(6.51965265029488,2.97784064076311,4.3179783102547));
#20471=CARTESIAN_POINT('Ctrl Pts',(6.90731160615835,3.32036226588665,4.3874112209937));
#20472=CARTESIAN_POINT('Ctrl Pts',(7.09222688286471,3.74505003376669,4.4504132977241));
#20473=CARTESIAN_POINT('Ctrl Pts',(7.10782115128883,4.16075024918538,4.50700494135613));
#20474=CARTESIAN_POINT('Ctrl Pts',(6.97052740566525,4.55245635004197,4.56347583453787));
#20475=CARTESIAN_POINT('Ctrl Pts',(6.67052546791681,4.90147648347343,4.62607046576882));
#20476=CARTESIAN_POINT('Ctrl Pts',(6.20415451901187,5.11161960500053,4.6947175781965));
#20477=CARTESIAN_POINT('Ctrl Pts',(5.64985527632065,5.06959112861472,4.76932506255945));
#20478=CARTESIAN_POINT('Ctrl Pts',(5.22368169854351,4.79395491895654,4.83741708200183));
#20479=CARTESIAN_POINT('Ctrl Pts',(4.98333509090071,4.40998685933077,4.899080077899));
#20480=CARTESIAN_POINT('Ctrl Pts',(4.88112298760244,3.87728182744366,4.97281135437488));
#20481=CARTESIAN_POINT('Ctrl Pts',(5.14030112762427,3.21712419472211,5.0644324068338));
#20482=CARTESIAN_POINT('Ctrl Pts',(5.90290458769374,2.85143281828595,5.17348771964845));
#20483=CARTESIAN_POINT('Ctrl Pts',(6.7026863026727,3.09982654772101,5.28157907216558));
#20484=CARTESIAN_POINT('Ctrl Pts',(7.11632239026351,3.81923483315095,5.38866562056333));
#20485=CARTESIAN_POINT('Ctrl Pts',(6.93207706426345,4.61994543349928,5.49470496192847));
#20486=CARTESIAN_POINT('Ctrl Pts',(6.25865467588588,5.07694576222689,5.59967634800426));
#20487=CARTESIAN_POINT('Ctrl Pts',(5.64053245488443,4.9819883712827,5.68046976345486));
#20488=CARTESIAN_POINT('Ctrl Pts',(5.30862714732133,4.72895402426325,5.73778470389805));
#20489=CARTESIAN_POINT('Ctrl Pts',(5.10096857886021,4.46928837163771,5.78347593827138));
#20490=CARTESIAN_POINT('Ctrl Pts',(4.97635818845021,4.06457032712951,5.84028308812804));
#20491=CARTESIAN_POINT('Ctrl Pts',(5.07699062710392,3.57040680685002,5.90797899550925));
#20492=CARTESIAN_POINT('Ctrl Pts',(5.39917799548324,3.18688187480847,5.9751998496335));
#20493=CARTESIAN_POINT('Ctrl Pts',(5.86231001106952,3.00572140277052,6.04195928029931));
#20494=CARTESIAN_POINT('Ctrl Pts',(6.31166975694251,3.06253707400158,6.10274005594962));
#20495=CARTESIAN_POINT('Ctrl Pts',(6.65277873543009,3.27774270105456,6.15767510739571));
#20496=CARTESIAN_POINT('Ctrl Pts',(6.94036467113044,3.66561745748298,6.22327456672061));
#20497=CARTESIAN_POINT('Ctrl Pts',(6.97826365807328,4.16716906221925,6.28840833804435));
#20498=CARTESIAN_POINT('Ctrl Pts',(6.75385045161079,4.58745250127139,6.35310168841968));
#20499=CARTESIAN_POINT('Ctrl Pts',(6.48522195348155,4.81896893074317,6.40141126646841));
#20500=CARTESIAN_POINT('Ctrl Pts',(6.15118675445815,4.93547873015213,6.44952021848864));
#20501=CARTESIAN_POINT('Ctrl Pts',(5.74056866270979,4.92033083741976,6.50542272631611));
#20502=CARTESIAN_POINT('Ctrl Pts',(5.32259389275759,4.68935725542832,6.56901537249866));
#20503=CARTESIAN_POINT('Ctrl Pts',(5.06421926497528,4.22100075031634,6.64018121519376));
#20504=CARTESIAN_POINT('Ctrl Pts',(5.08957030502715,3.77859543443293,6.69921364506262));
#20505=CARTESIAN_POINT('Ctrl Pts',(5.24759441716036,3.47372752194448,6.7462851377338));
#20506=CARTESIAN_POINT('Ctrl Pts',(5.44359092682464,3.26621147785527,6.78543652559592));
#20507=CARTESIAN_POINT('Ctrl Pts',(5.72292581228413,3.11861363079258,6.82841660268829));
#20508=CARTESIAN_POINT('Ctrl Pts',(6.06449785856132,3.08022887054951,6.87520054940006));
#20509=CARTESIAN_POINT('Ctrl Pts',(6.45141807695574,3.18362516656423,6.92968357040903));
#20510=CARTESIAN_POINT('Ctrl Pts',(6.79954021450763,3.4944566237918,6.99184376751914));
#20511=CARTESIAN_POINT('Ctrl Pts',(6.94455257369293,3.99851035174955,7.06165121796002));
#20512=CARTESIAN_POINT('Ctrl Pts',(6.79951881801366,4.50175945009174,7.13139176275215));
#20513=CARTESIAN_POINT('Ctrl Pts',(6.40906206282621,4.85072232716315,7.20110863853789));
#20514=CARTESIAN_POINT('Ctrl Pts',(5.89265231009902,4.93850009239064,7.27085083928631));
#20515=CARTESIAN_POINT('Ctrl Pts',(5.40816505578386,4.73793399235652,7.34066464993027));
#20516=CARTESIAN_POINT('Ctrl Pts',(5.10409736643278,4.30964140293706,7.41059704735086));
#20517=CARTESIAN_POINT('Ctrl Pts',(5.07438096238868,3.78399512770708,7.480693774379));
#20518=CARTESIAN_POINT('Ctrl Pts',(5.32959988196191,3.32170635411574,7.55099980642353));
#20519=CARTESIAN_POINT('Ctrl Pts',(5.79329351323159,3.06510017082497,7.62155879145399));
#20520=CARTESIAN_POINT('Ctrl Pts',(6.32465269238523,3.09460440832685,7.69241292590983));
#20521=CARTESIAN_POINT('Ctrl Pts',(6.76095436771159,3.40371072785635,7.76360261334252));
#20522=CARTESIAN_POINT('Ctrl Pts',(6.96703348947777,3.90014635488385,7.83516634058253));
#20523=CARTESIAN_POINT('Ctrl Pts',(6.87694103922925,4.43317690107195,7.90714028815697));
#20524=CARTESIAN_POINT('Ctrl Pts',(6.51483692341746,4.83908730724853,7.97955847764587));
#20525=CARTESIAN_POINT('Ctrl Pts',(5.98892532229963,4.9911480385519,8.05245175217812));
#20526=CARTESIAN_POINT('Ctrl Pts',(5.4589113285666,4.83908223472626,8.1258494649861));
#20527=CARTESIAN_POINT('Ctrl Pts',(5.10244841999796,4.44070302191148,8.197037283211));
#20528=CARTESIAN_POINT('Ctrl Pts',(5.00033453276715,3.93733852849481,8.26597109598537));
#20529=CARTESIAN_POINT('Ctrl Pts',(5.14639892975264,3.4630761983191,8.33258741168281));
#20530=CARTESIAN_POINT('Ctrl Pts',(5.47388873341462,3.1429125424487,8.39407540385829));
#20531=CARTESIAN_POINT('Ctrl Pts',(5.8641715122147,3.00649199677749,8.45031883640512));
#20532=CARTESIAN_POINT('Ctrl Pts',(6.23779892120356,3.02015709538156,8.50120513376291));
#20533=CARTESIAN_POINT('Ctrl Pts',(6.58242657954577,3.17041697479611,8.55235638725947));
#20534=CARTESIAN_POINT('Ctrl Pts',(6.84978347686345,3.43748813370884,8.60378217840298));
#20535=CARTESIAN_POINT('Ctrl Pts',(7.0018999972382,3.78564550978687,8.65547994429953));
#20536=CARTESIAN_POINT('Ctrl Pts',(7.01637209912577,4.16729382612512,8.70744988502598));
#20537=CARTESIAN_POINT('Ctrl Pts',(6.88975286292201,4.52974165060038,8.75969157924526));
#20538=CARTESIAN_POINT('Ctrl Pts',(6.63816518893249,4.82237901608623,8.81220378523025));
#20539=CARTESIAN_POINT('Ctrl Pts',(6.29530728381445,5.00379685458895,8.86498461008222));
#20540=CARTESIAN_POINT('Ctrl Pts',(5.90791617233848,5.0476255667439,8.91803141474409));
#20541=CARTESIAN_POINT('Ctrl Pts',(5.52943004553465,4.94639930136838,8.97134091897946));
#20542=CARTESIAN_POINT('Ctrl Pts',(5.21253131321036,4.71274027298687,9.02490904697504));
#20543=CARTESIAN_POINT('Ctrl Pts',(5.00195558202741,4.37791279978642,9.07873127653999));
#20544=CARTESIAN_POINT('Ctrl Pts',(4.92780662503539,3.98740302026396,9.1328019080889));
#20545=CARTESIAN_POINT('Ctrl Pts',(5.00203131662118,3.59525436515709,9.18711575654073));
#20546=CARTESIAN_POINT('Ctrl Pts',(5.23859924290997,3.21769111160157,9.24772564338878));
#20547=CARTESIAN_POINT('Ctrl Pts',(5.6577405937534,2.94654595863672,9.31472306283699));
#20548=CARTESIAN_POINT('Ctrl Pts',(6.2036069027209,2.90560752486482,9.38820031602263));
#20549=CARTESIAN_POINT('Ctrl Pts',(6.72629572804827,3.14075483532117,9.46511861157904));
#20550=CARTESIAN_POINT('Ctrl Pts',(7.07628215733169,3.63287033183077,9.54550944492924));
#20551=CARTESIAN_POINT('Ctrl Pts',(7.11197851063729,4.26218483646211,9.62939466251746));
#20552=CARTESIAN_POINT('Ctrl Pts',(6.80612080116325,4.81633859449139,9.71364494828372));
#20553=CARTESIAN_POINT('Ctrl Pts',(6.25008049897017,5.12402461510688,9.7982215811763));
#20554=CARTESIAN_POINT('Ctrl Pts',(5.6134379987664,5.08853941337726,9.88308356774128));
#20555=CARTESIAN_POINT('Ctrl Pts',(5.09177315554737,4.71869231988539,9.96818842663893));
#20556=CARTESIAN_POINT('Ctrl Pts',(4.84630700308618,4.12658530064136,10.0534921586305));
#20557=CARTESIAN_POINT('Ctrl Pts',(4.95372152652599,3.49350492422017,10.1389496180362));
#20558=CARTESIAN_POINT('Ctrl Pts',(5.38206851630237,3.01403467231803,10.2245147568725));
#20559=CARTESIAN_POINT('Ctrl Pts',(6.00030951953899,2.8358711302214,10.3101408922417));
#20560=CARTESIAN_POINT('Ctrl Pts',(6.61866596499084,3.01401901259021,10.3957809807524));
#20561=CARTESIAN_POINT('Ctrl Pts',(7.04725829779998,3.49369742862853,10.4813878741368));
#20562=CARTESIAN_POINT('Ctrl Pts',(7.15479989009825,4.12729588111062,10.5669146583618));
#20563=CARTESIAN_POINT('Ctrl Pts',(6.90907550905602,4.72009892225302,10.6523148500976));
#20564=CARTESIAN_POINT('Ctrl Pts',(6.38664410339373,5.09051877209641,10.7375427426944));
#20565=CARTESIAN_POINT('Ctrl Pts',(5.74882898183749,5.1260709263418,10.82255355924));
#20566=CARTESIAN_POINT('Ctrl Pts',(5.19158297309713,4.81774319749305,10.9073039912296));
#20567=CARTESIAN_POINT('Ctrl Pts',(4.88491211716783,4.26215901548285,10.9917518139848));
#20568=CARTESIAN_POINT('Ctrl Pts',(4.92071110615179,3.63115782136658,11.0758574895253));
#20569=CARTESIAN_POINT('Ctrl Pts',(5.28508855785184,3.11823615335598,11.1595814256275));
#20570=CARTESIAN_POINT('Ctrl Pts',(5.86358545423481,2.87909939337298,11.2428907919858));
#20571=CARTESIAN_POINT('Ctrl Pts',(6.47726426997602,2.98368077187355,11.3257449258384));
#20572=CARTESIAN_POINT('Ctrl Pts',(6.93842416474904,3.39673555851352,11.4081288318684));
#20573=CARTESIAN_POINT('Ctrl Pts',(7.05150181122087,3.79037870851095,11.4626969504405));
#20574=CARTESIAN_POINT('Ctrl Pts',(7.05152835862377,3.98757933451432,11.489920840408));
#20575=CARTESIAN_POINT('Ctrl Pts',(6.99999815899373,4.01367547347479,2.60093950625072));
#20576=CARTESIAN_POINT('Ctrl Pts',(6.99997288064589,4.20144961727953,2.62686205390015));
#20577=CARTESIAN_POINT('Ctrl Pts',(6.89230845853935,4.57620131355266,2.67882572810781));
#20578=CARTESIAN_POINT('Ctrl Pts',(6.45268902055693,4.97011892113672,2.75738771144581));
#20579=CARTESIAN_POINT('Ctrl Pts',(5.86669155617951,5.07009441973235,2.83651805910941));
#20580=CARTESIAN_POINT('Ctrl Pts',(5.31323924231124,4.84148977638369,2.91622570222972));
#20581=CARTESIAN_POINT('Ctrl Pts',(4.96382442320151,4.34995448969575,2.99649058141579));
#20582=CARTESIAN_POINT('Ctrl Pts',(4.92922815468166,3.74381008719936,3.07730076310524));
#20583=CARTESIAN_POINT('Ctrl Pts',(5.22433988671615,3.20870475874992,3.15863604084508));
#20584=CARTESIAN_POINT('Ctrl Pts',(5.76222017520179,2.91082295270622,3.24047540691231));
#20585=CARTESIAN_POINT('Ctrl Pts',(6.37972244802771,2.94499376197989,3.3227938596108));
#20586=CARTESIAN_POINT('Ctrl Pts',(6.88714214280083,3.30444617999842,3.40556405334158));
#20587=CARTESIAN_POINT('Ctrl Pts',(7.1267179261553,3.88170395597293,3.48875576611263));
#20588=CARTESIAN_POINT('Ctrl Pts',(7.02193956541344,4.50081591971197,3.57233637082151));
#20589=CARTESIAN_POINT('Ctrl Pts',(6.60200309921583,4.97124649007052,3.65627092163634));
#20590=CARTESIAN_POINT('Ctrl Pts',(5.99391816782283,5.1467637293928,3.74052239101179));
#20591=CARTESIAN_POINT('Ctrl Pts',(5.38351410020794,4.97125258500565,3.82505187835831));
#20592=CARTESIAN_POINT('Ctrl Pts',(4.97495278641361,4.51407471129711,3.90667930564871));
#20593=CARTESIAN_POINT('Ctrl Pts',(4.85890493436876,3.9395318134167,3.98533819655606));
#20594=CARTESIAN_POINT('Ctrl Pts',(5.0248445336464,3.40104453051283,4.06097495851984));
#20595=CARTESIAN_POINT('Ctrl Pts',(5.42877344681216,3.00706135834947,4.13670514776413));
#20596=CARTESIAN_POINT('Ctrl Pts',(5.97224138292893,2.85377277882407,4.21249751166765));
#20597=CARTESIAN_POINT('Ctrl Pts',(6.52306794486814,2.97976887786423,4.28832050304671));
#20598=CARTESIAN_POINT('Ctrl Pts',(6.911106619782,3.32248792481664,4.35782394345616));
#20599=CARTESIAN_POINT('Ctrl Pts',(7.09651656274147,3.74815778477591,4.4209850314008));
#20600=CARTESIAN_POINT('Ctrl Pts',(7.11222142726568,4.16541427135673,4.47779829351342));
#20601=CARTESIAN_POINT('Ctrl Pts',(6.97427650626816,4.55914085431083,4.53456660987697));
#20602=CARTESIAN_POINT('Ctrl Pts',(6.6723790417336,4.91046294860728,4.59757802409045));
#20603=CARTESIAN_POINT('Ctrl Pts',(6.20229995228089,5.12240612151564,4.66678931423933));
#20604=CARTESIAN_POINT('Ctrl Pts',(5.6425500433818,5.08009523000915,4.74213609069821));
#20605=CARTESIAN_POINT('Ctrl Pts',(5.21136094690014,4.8013569526932,4.8110335703418));
#20606=CARTESIAN_POINT('Ctrl Pts',(4.96782069609662,4.41239190726546,4.87351124705845));
#20607=CARTESIAN_POINT('Ctrl Pts',(4.86407127402864,3.87207825314686,4.94830807657783));
#20608=CARTESIAN_POINT('Ctrl Pts',(5.12715288076494,3.20107434287668,5.041444793684));
#20609=CARTESIAN_POINT('Ctrl Pts',(5.90376531288412,2.82823955973182,5.15254762811187));
#20610=CARTESIAN_POINT('Ctrl Pts',(6.72029013273465,3.08146453910134,5.2629101070658));
#20611=CARTESIAN_POINT('Ctrl Pts',(7.14364665428008,3.81715099008766,5.37246078991918));
#20612=CARTESIAN_POINT('Ctrl Pts',(6.9551205530812,4.63769652624648,5.4811367937548));
#20613=CARTESIAN_POINT('Ctrl Pts',(6.2641024490546,5.1069317667711,5.5888844628491));
#20614=CARTESIAN_POINT('Ctrl Pts',(5.62881174521816,5.00949357808685,5.67193196549233));
#20615=CARTESIAN_POINT('Ctrl Pts',(5.2874560242671,4.74926815537235,5.73087908447157));
#20616=CARTESIAN_POINT('Ctrl Pts',(5.07381541095866,4.48213637560843,5.77788659685938));
#20617=CARTESIAN_POINT('Ctrl Pts',(4.94552168624609,4.06557538718633,5.83636209008294));
#20618=CARTESIAN_POINT('Ctrl Pts',(5.04911869155687,3.55670415977292,5.90607316299982));
#20619=CARTESIAN_POINT('Ctrl Pts',(5.38099173791495,3.16160536520236,5.97532164753646));
#20620=CARTESIAN_POINT('Ctrl Pts',(5.85816561666817,2.97493727370523,6.04410657341625));
#20621=CARTESIAN_POINT('Ctrl Pts',(6.32119024886796,3.03347138881056,6.1067356435835));
#20622=CARTESIAN_POINT('Ctrl Pts',(6.67264815667528,3.25520245847479,6.16333652453463));
#20623=CARTESIAN_POINT('Ctrl Pts',(6.9689172446974,3.65479400388877,6.23091649769543));
#20624=CARTESIAN_POINT('Ctrl Pts',(7.0079089842411,4.17131843581214,6.29799027327548));
#20625=CARTESIAN_POINT('Ctrl Pts',(6.77691391923214,4.60388596675421,6.36457330679182));
#20626=CARTESIAN_POINT('Ctrl Pts',(6.50054973430609,4.84205531318333,6.414270318429));
#20627=CARTESIAN_POINT('Ctrl Pts',(6.15708960805529,4.96183696463414,6.46373244636263));
#20628=CARTESIAN_POINT('Ctrl Pts',(5.73515865256543,4.94625066250657,6.52117144063107));
#20629=CARTESIAN_POINT('Ctrl Pts',(5.30609465295405,4.70907742816445,6.5864458994691));
#20630=CARTESIAN_POINT('Ctrl Pts',(5.04126574291307,4.22881801076535,6.65940509117474));
#20631=CARTESIAN_POINT('Ctrl Pts',(5.06730780646012,3.7758858483265,6.71983222415362));
#20632=CARTESIAN_POINT('Ctrl Pts',(5.22892555890349,3.46412922360998,6.7679659145206));
#20633=CARTESIAN_POINT('Ctrl Pts',(5.4292015128227,3.25210405867328,6.80796630929891));
#20634=CARTESIAN_POINT('Ctrl Pts',(5.71433691472614,3.10148200562693,6.85183024183257));
#20635=CARTESIAN_POINT('Ctrl Pts',(6.06256514105404,3.06238687711817,6.89952195897341));
#20636=CARTESIAN_POINT('Ctrl Pts',(6.4564976195634,3.16770820022483,6.95498839068538));
#20637=CARTESIAN_POINT('Ctrl Pts',(6.8102288164166,3.48372159458398,7.01814871427154));
#20638=CARTESIAN_POINT('Ctrl Pts',(6.95714247630162,3.9949743218129,7.08893288176131));
#20639=CARTESIAN_POINT('Ctrl Pts',(6.81021696910949,4.50416338125004,7.1594866624322));
#20640=CARTESIAN_POINT('Ctrl Pts',(6.41591912974157,4.85632155826513,7.22985222666365));
#20641=CARTESIAN_POINT('Ctrl Pts',(5.89581150258709,4.9445435848153,7.30007283488175));
#20642=CARTESIAN_POINT('Ctrl Pts',(5.4091541149686,4.74288106481787,7.37019262264602));
#20643=CARTESIAN_POINT('Ctrl Pts',(5.1045916955003,4.31357351873737,7.4402563254929));
#20644=CARTESIAN_POINT('Ctrl Pts',(5.07507074796588,3.78812027671986,7.51030900575102));
#20645=CARTESIAN_POINT('Ctrl Pts',(5.32971571962661,3.32725097083008,7.58039577698861));
#20646=CARTESIAN_POINT('Ctrl Pts',(5.79102376728976,3.07217291555275,7.65056157443439));
#20647=CARTESIAN_POINT('Ctrl Pts',(6.31826217852957,3.10162768020774,7.72085085716367));
#20648=CARTESIAN_POINT('Ctrl Pts',(6.75007083293795,3.40776502742426,7.79130734598018));
#20649=CARTESIAN_POINT('Ctrl Pts',(6.95345754831281,3.89815513784294,7.86197377424134));
#20650=CARTESIAN_POINT('Ctrl Pts',(6.86450758322969,4.42345798565047,7.9328916442996));
#20651=CARTESIAN_POINT('Ctrl Pts',(6.50825373195115,4.82258144361629,8.00410096577401));
#20652=CARTESIAN_POINT('Ctrl Pts',(5.99196133471143,4.97171282731416,8.07564000535001));
#20653=CARTESIAN_POINT('Ctrl Pts',(5.47264846544098,4.82257977354425,8.14754510597589));
#20654=CARTESIAN_POINT('Ctrl Pts',(5.12402089676511,4.43277938176583,8.21717246163365));
#20655=CARTESIAN_POINT('Ctrl Pts',(5.02434526751946,3.94102818280025,8.28449961898673));
#20656=CARTESIAN_POINT('Ctrl Pts',(5.16694197219437,3.47827882962972,8.34949563910625));
#20657=CARTESIAN_POINT('Ctrl Pts',(5.48619587513468,3.16623898773365,8.40942447363167));
#20658=CARTESIAN_POINT('Ctrl Pts',(5.86631955340104,3.03340212556353,8.46419547601151));
#20659=CARTESIAN_POINT('Ctrl Pts',(6.22999033724363,3.04672408117636,8.5137197912885));
#20660=CARTESIAN_POINT('Ctrl Pts',(6.56525962631825,3.19292643023923,8.5634804916257));
#20661=CARTESIAN_POINT('Ctrl Pts',(6.82522778577244,3.45264122124887,8.61348288970028));
#20662=CARTESIAN_POINT('Ctrl Pts',(6.97307814435936,3.7910761621246,8.66373168303779));
#20663=CARTESIAN_POINT('Ctrl Pts',(6.98712736643486,4.16195247500926,8.71423091450252));
#20664=CARTESIAN_POINT('Ctrl Pts',(6.86409623902891,4.5140922960367,8.76498396821101));
#20665=CARTESIAN_POINT('Ctrl Pts',(6.61968565405262,4.79836651831856,8.81599356006379));
#20666=CARTESIAN_POINT('Ctrl Pts',(6.28663324217223,4.97458782653242,8.86726173278701));
#20667=CARTESIAN_POINT('Ctrl Pts',(5.9103163648716,5.01715912899264,8.91878984727219));
#20668=CARTESIAN_POINT('Ctrl Pts',(5.5426151162157,4.91881558382611,8.97057858184767));
#20669=CARTESIAN_POINT('Ctrl Pts',(5.2346932137367,4.69177671709244,9.02262792714338));
#20670=CARTESIAN_POINT('Ctrl Pts',(5.03002927873253,4.36635777160092,9.07493719269484));
#20671=CARTESIAN_POINT('Ctrl Pts',(4.95793528493379,3.98670141138964,9.12750499446544));
#20672=CARTESIAN_POINT('Ctrl Pts',(5.03011221582078,3.60530312678215,9.18032928985668));
#20673=CARTESIAN_POINT('Ctrl Pts',(5.26028491013977,3.23792219176526,9.23930487837506));
#20674=CARTESIAN_POINT('Ctrl Pts',(5.66833767471456,2.97390330572424,9.30453505298122));
#20675=CARTESIAN_POINT('Ctrl Pts',(6.20020835504347,2.93396150339657,9.37613052320119));
#20676=CARTESIAN_POINT('Ctrl Pts',(6.70998344550478,3.16323515745987,9.45115011118038));
#20677=CARTESIAN_POINT('Ctrl Pts',(7.05174463296735,3.64363058779886,9.52964181253653));
#20678=CARTESIAN_POINT('Ctrl Pts',(7.08674491429888,4.25878461683797,9.61164803498578));
#20679=CARTESIAN_POINT('Ctrl Pts',(6.78746221281555,4.80126791369132,9.69412424256602));
#20680=CARTESIAN_POINT('Ctrl Pts',(6.24245359179364,5.10299460367291,9.77704205650278));
#20681=CARTESIAN_POINT('Ctrl Pts',(5.617389337803,5.06829072683056,9.86037045574097));
#20682=CARTESIAN_POINT('Ctrl Pts',(5.10428990247565,4.70469241242162,9.94407602255943));
#20683=CARTESIAN_POINT('Ctrl Pts',(4.86233610468105,4.12145238678417,10.0281230884956));
#20684=CARTESIAN_POINT('Ctrl Pts',(4.96818752346366,3.49664100367693,10.1124739581892));
#20685=CARTESIAN_POINT('Ctrl Pts',(5.39158733307429,3.02246211865203,10.197089152739));
#20686=CARTESIAN_POINT('Ctrl Pts',(6.00398991824946,2.84580444666258,10.2819276236503));
#20687=CARTESIAN_POINT('Ctrl Pts',(6.61780477214459,3.0224619351938,10.3669470022194));
#20688=CARTESIAN_POINT('Ctrl Pts',(7.04420003577297,3.49941215707345,10.4521038303345));
#20689=CARTESIAN_POINT('Ctrl Pts',(7.15155414725,4.13081128487796,10.5373538665558));
#20690=CARTESIAN_POINT('Ctrl Pts',(6.90634183228622,4.72286458915024,10.6226522963591));
#20691=CARTESIAN_POINT('Ctrl Pts',(6.38367034420738,5.09368398946472,10.7079540131199));
#20692=CARTESIAN_POINT('Ctrl Pts',(5.74412845724406,5.12951897848491,10.7932138931513));
#20693=CARTESIAN_POINT('Ctrl Pts',(5.18413119725411,4.81987766303419,10.8783870658711));
#20694=CARTESIAN_POINT('Ctrl Pts',(4.8752129919825,4.26058851376116,10.9634291554075));
#20695=CARTESIAN_POINT('Ctrl Pts',(4.91115871222138,3.62399076997319,11.0482965295163));
#20696=CARTESIAN_POINT('Ctrl Pts',(5.27935908785992,3.10540850794678,11.1329466617017));
#20697=CARTESIAN_POINT('Ctrl Pts',(5.86521072908837,2.86304864268273,11.2173381122335));
#20698=CARTESIAN_POINT('Ctrl Pts',(6.48796989668153,2.969020134583,11.3014313415043));
#20699=CARTESIAN_POINT('Ctrl Pts',(6.95689206969945,3.38875839075872,11.3851878190745));
#20700=CARTESIAN_POINT('Ctrl Pts',(7.07219562678887,3.7896496622666,11.4407823887692));
#20701=CARTESIAN_POINT('Ctrl Pts',(7.07222266979222,3.99053173007441,11.4685145081913));
#20702=CARTESIAN_POINT('',(6.99999815899373,4.01367547347479,2.60093950625072));
#20703=CARTESIAN_POINT('Origin',(7.,4.,2.7));
#20704=CARTESIAN_POINT('',(7.07222266979222,3.99053173007441,11.4685145081913));
#20705=CARTESIAN_POINT('Ctrl Pts',(6.99999815899373,4.01367547347479,2.60093950625072));
#20706=CARTESIAN_POINT('Ctrl Pts',(6.99997288064589,4.20144961727953,2.62686205390015));
#20707=CARTESIAN_POINT('Ctrl Pts',(6.89230845853935,4.57620131355266,2.67882572810781));
#20708=CARTESIAN_POINT('Ctrl Pts',(6.45268902055693,4.97011892113672,2.75738771144581));
#20709=CARTESIAN_POINT('Ctrl Pts',(5.86669155617951,5.07009441973235,2.83651805910941));
#20710=CARTESIAN_POINT('Ctrl Pts',(5.31323924231124,4.84148977638369,2.91622570222972));
#20711=CARTESIAN_POINT('Ctrl Pts',(4.96382442320151,4.34995448969575,2.99649058141579));
#20712=CARTESIAN_POINT('Ctrl Pts',(4.92922815468166,3.74381008719936,3.07730076310524));
#20713=CARTESIAN_POINT('Ctrl Pts',(5.22433988671615,3.20870475874992,3.15863604084508));
#20714=CARTESIAN_POINT('Ctrl Pts',(5.76222017520179,2.91082295270622,3.24047540691231));
#20715=CARTESIAN_POINT('Ctrl Pts',(6.37972244802771,2.94499376197989,3.3227938596108));
#20716=CARTESIAN_POINT('Ctrl Pts',(6.88714214280083,3.30444617999842,3.40556405334158));
#20717=CARTESIAN_POINT('Ctrl Pts',(7.1267179261553,3.88170395597293,3.48875576611263));
#20718=CARTESIAN_POINT('Ctrl Pts',(7.02193956541344,4.50081591971197,3.57233637082151));
#20719=CARTESIAN_POINT('Ctrl Pts',(6.60200309921583,4.97124649007052,3.65627092163634));
#20720=CARTESIAN_POINT('Ctrl Pts',(5.99391816782283,5.1467637293928,3.74052239101179));
#20721=CARTESIAN_POINT('Ctrl Pts',(5.38351410020794,4.97125258500565,3.82505187835831));
#20722=CARTESIAN_POINT('Ctrl Pts',(4.97495278641361,4.51407471129711,3.90667930564871));
#20723=CARTESIAN_POINT('Ctrl Pts',(4.85890493436876,3.9395318134167,3.98533819655606));
#20724=CARTESIAN_POINT('Ctrl Pts',(5.0248445336464,3.40104453051283,4.06097495851984));
#20725=CARTESIAN_POINT('Ctrl Pts',(5.42877344681216,3.00706135834947,4.13670514776413));
#20726=CARTESIAN_POINT('Ctrl Pts',(5.97224138292893,2.85377277882407,4.21249751166765));
#20727=CARTESIAN_POINT('Ctrl Pts',(6.52306794486814,2.97976887786423,4.28832050304671));
#20728=CARTESIAN_POINT('Ctrl Pts',(6.911106619782,3.32248792481664,4.35782394345616));
#20729=CARTESIAN_POINT('Ctrl Pts',(7.09651656274147,3.74815778477591,4.4209850314008));
#20730=CARTESIAN_POINT('Ctrl Pts',(7.11222142726568,4.16541427135673,4.47779829351342));
#20731=CARTESIAN_POINT('Ctrl Pts',(6.97427650626816,4.55914085431083,4.53456660987697));
#20732=CARTESIAN_POINT('Ctrl Pts',(6.6723790417336,4.91046294860728,4.59757802409045));
#20733=CARTESIAN_POINT('Ctrl Pts',(6.20229995228089,5.12240612151564,4.66678931423933));
#20734=CARTESIAN_POINT('Ctrl Pts',(5.6425500433818,5.08009523000915,4.74213609069821));
#20735=CARTESIAN_POINT('Ctrl Pts',(5.21136094690014,4.8013569526932,4.8110335703418));
#20736=CARTESIAN_POINT('Ctrl Pts',(4.96782069609662,4.41239190726546,4.87351124705845));
#20737=CARTESIAN_POINT('Ctrl Pts',(4.86407127402864,3.87207825314686,4.94830807657783));
#20738=CARTESIAN_POINT('Ctrl Pts',(5.12715288076494,3.20107434287668,5.041444793684));
#20739=CARTESIAN_POINT('Ctrl Pts',(5.90376531288412,2.82823955973182,5.15254762811187));
#20740=CARTESIAN_POINT('Ctrl Pts',(6.72029013273465,3.08146453910134,5.2629101070658));
#20741=CARTESIAN_POINT('Ctrl Pts',(7.14364665428008,3.81715099008766,5.37246078991918));
#20742=CARTESIAN_POINT('Ctrl Pts',(6.9551205530812,4.63769652624648,5.4811367937548));
#20743=CARTESIAN_POINT('Ctrl Pts',(6.2641024490546,5.1069317667711,5.5888844628491));
#20744=CARTESIAN_POINT('Ctrl Pts',(5.62881174521816,5.00949357808685,5.67193196549233));
#20745=CARTESIAN_POINT('Ctrl Pts',(5.2874560242671,4.74926815537235,5.73087908447157));
#20746=CARTESIAN_POINT('Ctrl Pts',(5.07381541095866,4.48213637560843,5.77788659685938));
#20747=CARTESIAN_POINT('Ctrl Pts',(4.94552168624609,4.06557538718633,5.83636209008294));
#20748=CARTESIAN_POINT('Ctrl Pts',(5.04911869155687,3.55670415977292,5.90607316299982));
#20749=CARTESIAN_POINT('Ctrl Pts',(5.38099173791495,3.16160536520236,5.97532164753646));
#20750=CARTESIAN_POINT('Ctrl Pts',(5.85816561666817,2.97493727370523,6.04410657341625));
#20751=CARTESIAN_POINT('Ctrl Pts',(6.32119024886796,3.03347138881056,6.1067356435835));
#20752=CARTESIAN_POINT('Ctrl Pts',(6.67264815667528,3.25520245847479,6.16333652453463));
#20753=CARTESIAN_POINT('Ctrl Pts',(6.9689172446974,3.65479400388877,6.23091649769543));
#20754=CARTESIAN_POINT('Ctrl Pts',(7.0079089842411,4.17131843581214,6.29799027327548));
#20755=CARTESIAN_POINT('Ctrl Pts',(6.77691391923214,4.60388596675421,6.36457330679182));
#20756=CARTESIAN_POINT('Ctrl Pts',(6.50054973430609,4.84205531318333,6.414270318429));
#20757=CARTESIAN_POINT('Ctrl Pts',(6.15708960805529,4.96183696463414,6.46373244636263));
#20758=CARTESIAN_POINT('Ctrl Pts',(5.73515865256543,4.94625066250657,6.52117144063107));
#20759=CARTESIAN_POINT('Ctrl Pts',(5.30609465295405,4.70907742816445,6.5864458994691));
#20760=CARTESIAN_POINT('Ctrl Pts',(5.04126574291307,4.22881801076535,6.65940509117474));
#20761=CARTESIAN_POINT('Ctrl Pts',(5.06730780646012,3.7758858483265,6.71983222415362));
#20762=CARTESIAN_POINT('Ctrl Pts',(5.22892555890349,3.46412922360998,6.7679659145206));
#20763=CARTESIAN_POINT('Ctrl Pts',(5.4292015128227,3.25210405867328,6.80796630929891));
#20764=CARTESIAN_POINT('Ctrl Pts',(5.71433691472614,3.10148200562693,6.85183024183257));
#20765=CARTESIAN_POINT('Ctrl Pts',(6.06256514105404,3.06238687711817,6.89952195897341));
#20766=CARTESIAN_POINT('Ctrl Pts',(6.4564976195634,3.16770820022483,6.95498839068538));
#20767=CARTESIAN_POINT('Ctrl Pts',(6.8102288164166,3.48372159458398,7.01814871427154));
#20768=CARTESIAN_POINT('Ctrl Pts',(6.95714247630162,3.9949743218129,7.08893288176131));
#20769=CARTESIAN_POINT('Ctrl Pts',(6.81021696910949,4.50416338125004,7.1594866624322));
#20770=CARTESIAN_POINT('Ctrl Pts',(6.41591912974157,4.85632155826513,7.22985222666365));
#20771=CARTESIAN_POINT('Ctrl Pts',(5.89581150258709,4.9445435848153,7.30007283488175));
#20772=CARTESIAN_POINT('Ctrl Pts',(5.4091541149686,4.74288106481787,7.37019262264602));
#20773=CARTESIAN_POINT('Ctrl Pts',(5.1045916955003,4.31357351873737,7.4402563254929));
#20774=CARTESIAN_POINT('Ctrl Pts',(5.07507074796588,3.78812027671986,7.51030900575102));
#20775=CARTESIAN_POINT('Ctrl Pts',(5.32971571962661,3.32725097083008,7.58039577698861));
#20776=CARTESIAN_POINT('Ctrl Pts',(5.79102376728976,3.07217291555275,7.65056157443439));
#20777=CARTESIAN_POINT('Ctrl Pts',(6.31826217852957,3.10162768020774,7.72085085716367));
#20778=CARTESIAN_POINT('Ctrl Pts',(6.75007083293795,3.40776502742426,7.79130734598018));
#20779=CARTESIAN_POINT('Ctrl Pts',(6.95345754831281,3.89815513784294,7.86197377424134));
#20780=CARTESIAN_POINT('Ctrl Pts',(6.86450758322969,4.42345798565047,7.9328916442996));
#20781=CARTESIAN_POINT('Ctrl Pts',(6.50825373195115,4.82258144361629,8.00410096577401));
#20782=CARTESIAN_POINT('Ctrl Pts',(5.99196133471143,4.97171282731416,8.07564000535001));
#20783=CARTESIAN_POINT('Ctrl Pts',(5.47264846544098,4.82257977354425,8.14754510597589));
#20784=CARTESIAN_POINT('Ctrl Pts',(5.12402089676511,4.43277938176583,8.21717246163365));
#20785=CARTESIAN_POINT('Ctrl Pts',(5.02434526751946,3.94102818280025,8.28449961898673));
#20786=CARTESIAN_POINT('Ctrl Pts',(5.16694197219437,3.47827882962972,8.34949563910625));
#20787=CARTESIAN_POINT('Ctrl Pts',(5.48619587513468,3.16623898773365,8.40942447363167));
#20788=CARTESIAN_POINT('Ctrl Pts',(5.86631955340104,3.03340212556353,8.46419547601151));
#20789=CARTESIAN_POINT('Ctrl Pts',(6.22999033724363,3.04672408117636,8.5137197912885));
#20790=CARTESIAN_POINT('Ctrl Pts',(6.56525962631825,3.19292643023923,8.5634804916257));
#20791=CARTESIAN_POINT('Ctrl Pts',(6.82522778577244,3.45264122124887,8.61348288970028));
#20792=CARTESIAN_POINT('Ctrl Pts',(6.97307814435936,3.7910761621246,8.66373168303779));
#20793=CARTESIAN_POINT('Ctrl Pts',(6.98712736643486,4.16195247500926,8.71423091450252));
#20794=CARTESIAN_POINT('Ctrl Pts',(6.86409623902891,4.5140922960367,8.76498396821101));
#20795=CARTESIAN_POINT('Ctrl Pts',(6.61968565405262,4.79836651831856,8.81599356006379));
#20796=CARTESIAN_POINT('Ctrl Pts',(6.28663324217223,4.97458782653242,8.86726173278701));
#20797=CARTESIAN_POINT('Ctrl Pts',(5.9103163648716,5.01715912899264,8.91878984727219));
#20798=CARTESIAN_POINT('Ctrl Pts',(5.5426151162157,4.91881558382611,8.97057858184767));
#20799=CARTESIAN_POINT('Ctrl Pts',(5.2346932137367,4.69177671709244,9.02262792714338));
#20800=CARTESIAN_POINT('Ctrl Pts',(5.03002927873253,4.36635777160092,9.07493719269484));
#20801=CARTESIAN_POINT('Ctrl Pts',(4.95793528493379,3.98670141138964,9.12750499446544));
#20802=CARTESIAN_POINT('Ctrl Pts',(5.03011221582078,3.60530312678215,9.18032928985668));
#20803=CARTESIAN_POINT('Ctrl Pts',(5.26028491013977,3.23792219176526,9.23930487837506));
#20804=CARTESIAN_POINT('Ctrl Pts',(5.66833767471456,2.97390330572424,9.30453505298122));
#20805=CARTESIAN_POINT('Ctrl Pts',(6.20020835504347,2.93396150339657,9.37613052320119));
#20806=CARTESIAN_POINT('Ctrl Pts',(6.70998344550478,3.16323515745987,9.45115011118038));
#20807=CARTESIAN_POINT('Ctrl Pts',(7.05174463296735,3.64363058779886,9.52964181253653));
#20808=CARTESIAN_POINT('Ctrl Pts',(7.08674491429888,4.25878461683797,9.61164803498578));
#20809=CARTESIAN_POINT('Ctrl Pts',(6.78746221281555,4.80126791369132,9.69412424256602));
#20810=CARTESIAN_POINT('Ctrl Pts',(6.24245359179364,5.10299460367291,9.77704205650278));
#20811=CARTESIAN_POINT('Ctrl Pts',(5.617389337803,5.06829072683056,9.86037045574097));
#20812=CARTESIAN_POINT('Ctrl Pts',(5.10428990247565,4.70469241242162,9.94407602255943));
#20813=CARTESIAN_POINT('Ctrl Pts',(4.86233610468105,4.12145238678417,10.0281230884956));
#20814=CARTESIAN_POINT('Ctrl Pts',(4.96818752346366,3.49664100367693,10.1124739581892));
#20815=CARTESIAN_POINT('Ctrl Pts',(5.39158733307429,3.02246211865203,10.197089152739));
#20816=CARTESIAN_POINT('Ctrl Pts',(6.00398991824946,2.84580444666258,10.2819276236503));
#20817=CARTESIAN_POINT('Ctrl Pts',(6.61780477214459,3.0224619351938,10.3669470022194));
#20818=CARTESIAN_POINT('Ctrl Pts',(7.04420003577297,3.49941215707345,10.4521038303345));
#20819=CARTESIAN_POINT('Ctrl Pts',(7.15155414725,4.13081128487796,10.5373538665558));
#20820=CARTESIAN_POINT('Ctrl Pts',(6.90634183228622,4.72286458915024,10.6226522963591));
#20821=CARTESIAN_POINT('Ctrl Pts',(6.38367034420738,5.09368398946472,10.7079540131199));
#20822=CARTESIAN_POINT('Ctrl Pts',(5.74412845724406,5.12951897848491,10.7932138931513));
#20823=CARTESIAN_POINT('Ctrl Pts',(5.18413119725411,4.81987766303419,10.8783870658711));
#20824=CARTESIAN_POINT('Ctrl Pts',(4.8752129919825,4.26058851376116,10.9634291554075));
#20825=CARTESIAN_POINT('Ctrl Pts',(4.91115871222138,3.62399076997319,11.0482965295163));
#20826=CARTESIAN_POINT('Ctrl Pts',(5.27935908785992,3.10540850794678,11.1329466617017));
#20827=CARTESIAN_POINT('Ctrl Pts',(5.86521072908837,2.86304864268273,11.2173381122335));
#20828=CARTESIAN_POINT('Ctrl Pts',(6.48796989668153,2.969020134583,11.3014313415043));
#20829=CARTESIAN_POINT('Ctrl Pts',(6.95689206969945,3.38875839075872,11.3851878190745));
#20830=CARTESIAN_POINT('Ctrl Pts',(7.07219562678887,3.7896496622666,11.4407823887692));
#20831=CARTESIAN_POINT('Ctrl Pts',(7.07222266979222,3.99053173007441,11.4685145081913));
#20832=CARTESIAN_POINT('Origin',(7.,4.,11.4));
#20833=CARTESIAN_POINT('Origin',(7.,4.,11.4));
#20834=CARTESIAN_POINT('Origin',(7.,4.,2.7));
#22316=UNCERTAINTY_MEASURE_WITH_UNIT(LENGTH_MEASURE(0.001),#22395,
'DISTANCE_ACCURACY_VALUE',
'Maximum model space distance between geometric entities at asserted c
onnectivities');
#22343=UNCERTAINTY_MEASURE_WITH_UNIT(LENGTH_MEASURE(0.001),#22395,
'DISTANCE_ACCURACY_VALUE',
'Maximum model space distance between geometric entities at asserted c
onnectivities');
#22367=(
GEOMETRIC_REPRESENTATION_CONTEXT(3)
GLOBAL_UNCERTAINTY_ASSIGNED_CONTEXT((#22316))
GLOBAL_UNIT_ASSIGNED_CONTEXT((#22395,#22397,#22398))
REPRESENTATION_CONTEXT('','3D')
);
#22394=(
GEOMETRIC_REPRESENTATION_CONTEXT(3)
GLOBAL_UNCERTAINTY_ASSIGNED_CONTEXT((#22343))
GLOBAL_UNIT_ASSIGNED_CONTEXT((#22395,#22397,#22398))
REPRESENTATION_CONTEXT('','3D')
);
#22395=(
LENGTH_UNIT()
NAMED_UNIT(*)
SI_UNIT(.CENTI.,.METRE.)
);
#22397=(
NAMED_UNIT(*)
PLANE_ANGLE_UNIT()
SI_UNIT($,.RADIAN.)
);
#22398=(
NAMED_UNIT(*)
SI_UNIT($,.STERADIAN.)
SOLID_ANGLE_UNIT()
);
#22422=SHAPE_DEFINITION_REPRESENTATION(#22472,#22661);
#22472=PRODUCT_DEFINITION_SHAPE('',$,#22712);
#22661=SHAPE_REPRESENTATION('',(#10199),#22367);
#22688=PRODUCT_DEFINITION_CONTEXT('part definition',#22840,'design');
#22712=PRODUCT_DEFINITION('Installed compression spring (3)',
'Installed compression spring (3)',#22762,#22688);
#22762=PRODUCT_DEFINITION_FORMATION('',$,#22865);
#22840=APPLICATION_CONTEXT(
'Core Data for Automotive Mechanical Design Process');
#22841=PRODUCT_CONTEXT('part definition',#22840,'mechanical');
#22865=PRODUCT('Installed compression spring (3)',
'Installed compression spring (3)','Installed compression spring (3)',(#22841));
#22955=COLOUR_RGB('Grey',0.48,0.52,0.57);
#22956=FILL_AREA_STYLE_COLOUR('',#22955);
#22957=FILL_AREA_STYLE('',(#22956));
#22958=SURFACE_STYLE_FILL_AREA(#22957);
#22959=SURFACE_SIDE_STYLE('',(#22958));
#22960=SURFACE_STYLE_USAGE(.BOTH.,#22959);
#22961=PRESENTATION_STYLE_ASSIGNMENT((#22960));
ENDSEC;
END-ISO-10303-21;
